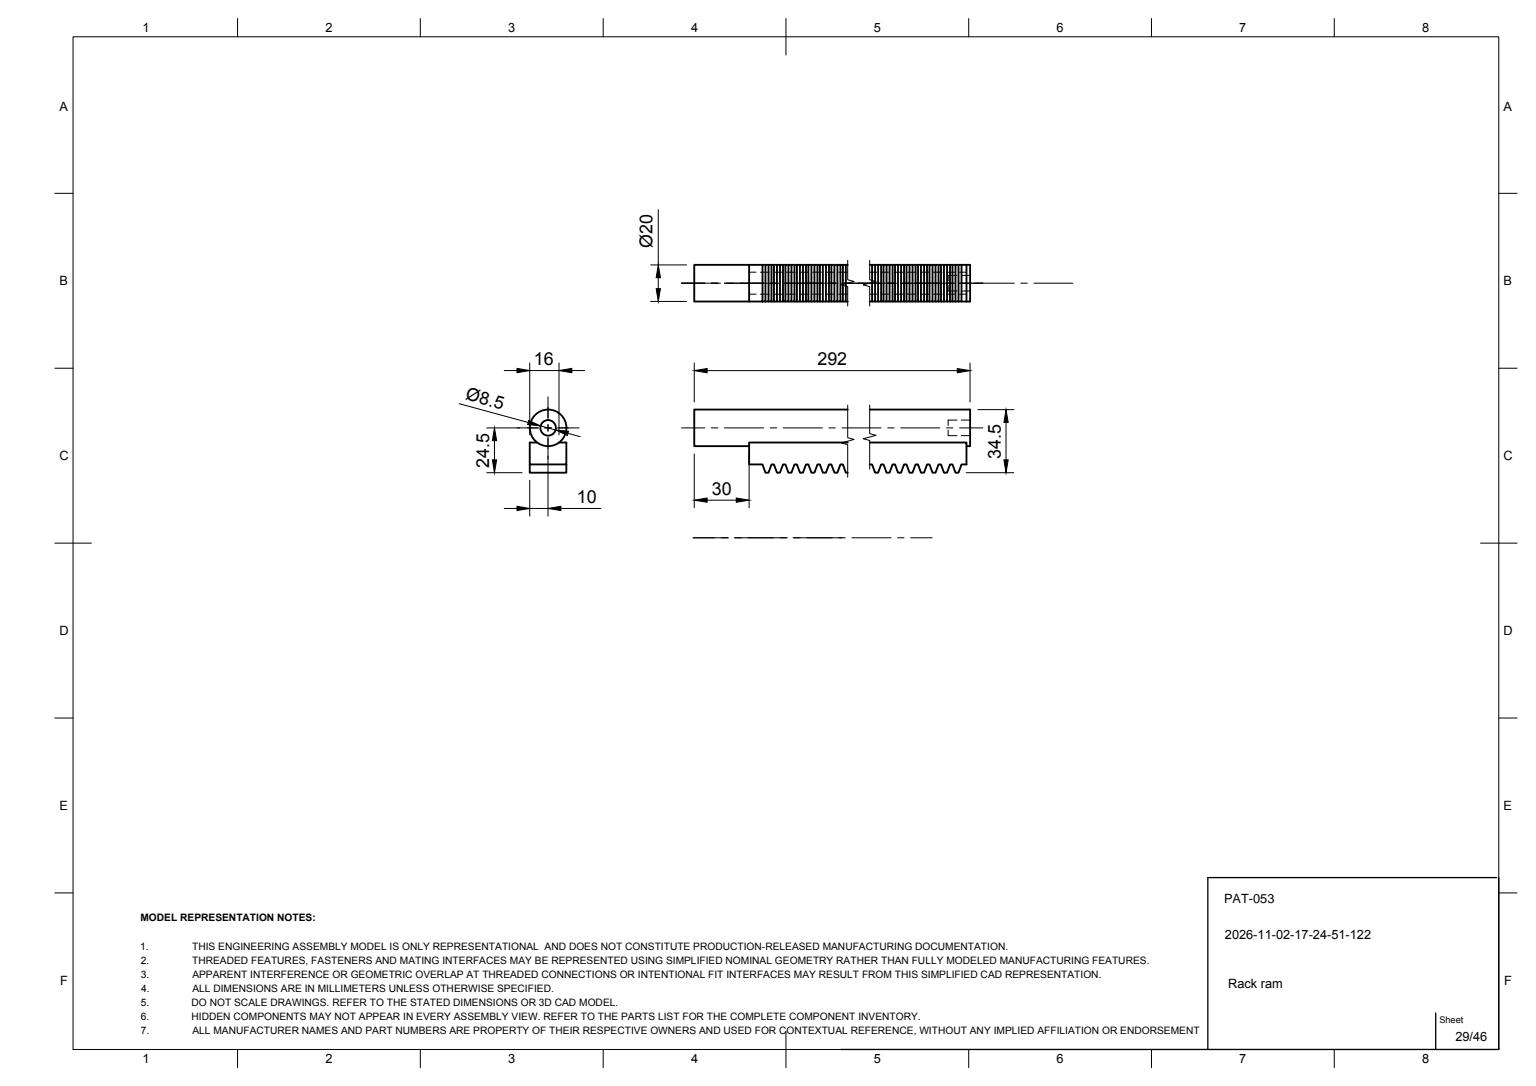
ISO-10303-21;
HEADER;
/* Generated by software containing ST-Developer
 * from STEP Tools, Inc. (www.steptools.com) 
 */

FILE_DESCRIPTION(
/* description */ ('Hand-operated arbor press'),
/* implementation_level */ '2;1');

FILE_NAME(
/* name */ 'Rack ram.step',
/* time_stamp */ '2026-10-28T03:25:25-07:00',
/* author */ (''),
/* organization */ (''),
/* preprocessor_version */ 'ST-DEVELOPER v20.2',
/* originating_system */ 'Autodesk Translation Framework v15.17.0.0',
/* authorisation */ '');

FILE_SCHEMA (('AUTOMOTIVE_DESIGN { 1 0 10303 214 3 1 1 }'));
ENDSEC;

DATA;
#10=MECHANICAL_DESIGN_GEOMETRIC_PRESENTATION_REPRESENTATION('',(#615),#32751);
#524=SHAPE_REPRESENTATION_RELATIONSHIP('SRR','None',#32955,#566);
#566=ADVANCED_BREP_SHAPE_REPRESENTATION('',(#662),#32729);
#615=STYLED_ITEM('',(#33228),#662);
#662=MANIFOLD_SOLID_BREP('Body1',#12514);
#812=FACE_BOUND('',#2561,.T.);
#1004=PLANE('',#13571);
#1005=PLANE('',#13572);
#1006=PLANE('',#13573);
#1007=PLANE('',#13574);
#1008=PLANE('',#13577);
#1009=PLANE('',#13580);
#1010=PLANE('',#13581);
#1011=PLANE('',#13582);
#1012=PLANE('',#13583);
#1013=PLANE('',#13584);
#1014=PLANE('',#13585);
#1015=PLANE('',#13586);
#1016=PLANE('',#13587);
#1017=PLANE('',#13588);
#1018=PLANE('',#13589);
#1019=PLANE('',#13590);
#1020=PLANE('',#13591);
#1021=PLANE('',#13592);
#1022=PLANE('',#13593);
#1023=PLANE('',#13594);
#1024=PLANE('',#13595);
#1025=PLANE('',#13596);
#1026=PLANE('',#13597);
#1027=PLANE('',#13598);
#1028=PLANE('',#13599);
#1029=PLANE('',#13600);
#1030=PLANE('',#13601);
#1031=PLANE('',#13602);
#1032=PLANE('',#13603);
#1033=PLANE('',#13604);
#1034=PLANE('',#13605);
#1035=PLANE('',#13606);
#1036=PLANE('',#13607);
#1037=PLANE('',#13608);
#1038=PLANE('',#13609);
#1039=PLANE('',#13610);
#1040=PLANE('',#13611);
#1041=PLANE('',#13612);
#1042=PLANE('',#13613);
#1043=PLANE('',#13614);
#1044=PLANE('',#13615);
#1045=PLANE('',#13616);
#1046=PLANE('',#13617);
#1047=PLANE('',#13618);
#1048=PLANE('',#13619);
#1049=PLANE('',#13620);
#1050=PLANE('',#13621);
#1051=PLANE('',#13622);
#1052=PLANE('',#13623);
#1053=PLANE('',#13624);
#1054=PLANE('',#13625);
#1055=PLANE('',#13626);
#1056=PLANE('',#13627);
#1057=PLANE('',#13628);
#1058=PLANE('',#13629);
#1059=PLANE('',#13630);
#1060=PLANE('',#13631);
#1061=PLANE('',#13632);
#1062=PLANE('',#13633);
#1063=PLANE('',#13634);
#1064=PLANE('',#13635);
#1065=PLANE('',#13636);
#1066=PLANE('',#13637);
#1067=PLANE('',#13638);
#1068=PLANE('',#13639);
#1069=PLANE('',#13640);
#1070=PLANE('',#13641);
#1071=PLANE('',#13642);
#1072=PLANE('',#13643);
#1073=PLANE('',#13644);
#1074=PLANE('',#13645);
#1075=PLANE('',#13646);
#1076=PLANE('',#13647);
#1077=PLANE('',#13648);
#1078=PLANE('',#13649);
#1079=PLANE('',#13650);
#1080=PLANE('',#13651);
#1081=PLANE('',#13652);
#1082=PLANE('',#13653);
#1083=PLANE('',#13654);
#1084=PLANE('',#13655);
#1085=PLANE('',#13656);
#1086=PLANE('',#13657);
#1087=PLANE('',#13658);
#1088=PLANE('',#13659);
#1089=PLANE('',#13660);
#1090=PLANE('',#13661);
#1091=PLANE('',#13662);
#1092=PLANE('',#13663);
#1093=PLANE('',#13664);
#1094=PLANE('',#13665);
#1095=PLANE('',#13666);
#1096=PLANE('',#13667);
#1097=PLANE('',#13668);
#1098=PLANE('',#13669);
#1099=PLANE('',#13670);
#1100=PLANE('',#13671);
#1101=PLANE('',#13672);
#1102=PLANE('',#13673);
#1103=PLANE('',#13674);
#1104=PLANE('',#13675);
#1105=PLANE('',#13676);
#1106=PLANE('',#13677);
#1107=PLANE('',#13678);
#1108=PLANE('',#13679);
#1109=PLANE('',#13680);
#1110=PLANE('',#13681);
#1111=PLANE('',#13682);
#1112=PLANE('',#13683);
#1113=PLANE('',#13684);
#1114=PLANE('',#13685);
#1115=PLANE('',#13686);
#1116=PLANE('',#13687);
#1117=PLANE('',#13688);
#1118=PLANE('',#13689);
#1119=PLANE('',#13690);
#1120=PLANE('',#13691);
#1121=PLANE('',#13692);
#1122=PLANE('',#13693);
#1123=PLANE('',#13694);
#1124=PLANE('',#13695);
#1125=PLANE('',#13696);
#1126=PLANE('',#13697);
#1127=PLANE('',#13698);
#1128=PLANE('',#13699);
#1129=PLANE('',#13700);
#1130=PLANE('',#13701);
#1131=PLANE('',#13702);
#1132=PLANE('',#13703);
#1133=PLANE('',#13704);
#1134=PLANE('',#13705);
#1135=PLANE('',#13706);
#1136=PLANE('',#13707);
#1137=PLANE('',#13708);
#1138=PLANE('',#13709);
#1139=PLANE('',#13710);
#1140=PLANE('',#13711);
#1141=PLANE('',#13712);
#1142=PLANE('',#13713);
#1143=PLANE('',#13714);
#1144=PLANE('',#13715);
#1145=PLANE('',#13716);
#1146=PLANE('',#13717);
#1147=PLANE('',#13718);
#1148=PLANE('',#13719);
#1149=PLANE('',#13720);
#1150=PLANE('',#13721);
#1151=PLANE('',#13722);
#1152=PLANE('',#13723);
#1153=PLANE('',#13724);
#1154=PLANE('',#13725);
#1155=PLANE('',#13726);
#1156=PLANE('',#13727);
#1157=PLANE('',#13728);
#1158=PLANE('',#13729);
#1159=PLANE('',#13730);
#1160=PLANE('',#13731);
#1161=PLANE('',#13732);
#1162=PLANE('',#13733);
#1163=PLANE('',#13734);
#1164=PLANE('',#13735);
#1165=PLANE('',#13736);
#1166=PLANE('',#13737);
#1167=PLANE('',#13738);
#1168=PLANE('',#13739);
#1169=PLANE('',#13740);
#1170=PLANE('',#13741);
#1171=PLANE('',#13742);
#1172=PLANE('',#13746);
#1173=PLANE('',#13747);
#1576=FACE_OUTER_BOUND('',#2389,.T.);
#1577=FACE_OUTER_BOUND('',#2390,.T.);
#1578=FACE_OUTER_BOUND('',#2391,.T.);
#1579=FACE_OUTER_BOUND('',#2392,.T.);
#1580=FACE_OUTER_BOUND('',#2393,.T.);
#1581=FACE_OUTER_BOUND('',#2394,.T.);
#1582=FACE_OUTER_BOUND('',#2395,.T.);
#1583=FACE_OUTER_BOUND('',#2396,.T.);
#1584=FACE_OUTER_BOUND('',#2397,.T.);
#1585=FACE_OUTER_BOUND('',#2398,.T.);
#1586=FACE_OUTER_BOUND('',#2399,.T.);
#1587=FACE_OUTER_BOUND('',#2400,.T.);
#1588=FACE_OUTER_BOUND('',#2401,.T.);
#1589=FACE_OUTER_BOUND('',#2402,.T.);
#1590=FACE_OUTER_BOUND('',#2403,.T.);
#1591=FACE_OUTER_BOUND('',#2404,.T.);
#1592=FACE_OUTER_BOUND('',#2405,.T.);
#1593=FACE_OUTER_BOUND('',#2406,.T.);
#1594=FACE_OUTER_BOUND('',#2407,.T.);
#1595=FACE_OUTER_BOUND('',#2408,.T.);
#1596=FACE_OUTER_BOUND('',#2409,.T.);
#1597=FACE_OUTER_BOUND('',#2410,.T.);
#1598=FACE_OUTER_BOUND('',#2411,.T.);
#1599=FACE_OUTER_BOUND('',#2412,.T.);
#1600=FACE_OUTER_BOUND('',#2413,.T.);
#1601=FACE_OUTER_BOUND('',#2414,.T.);
#1602=FACE_OUTER_BOUND('',#2415,.T.);
#1603=FACE_OUTER_BOUND('',#2416,.T.);
#1604=FACE_OUTER_BOUND('',#2417,.T.);
#1605=FACE_OUTER_BOUND('',#2418,.T.);
#1606=FACE_OUTER_BOUND('',#2419,.T.);
#1607=FACE_OUTER_BOUND('',#2420,.T.);
#1608=FACE_OUTER_BOUND('',#2421,.T.);
#1609=FACE_OUTER_BOUND('',#2422,.T.);
#1610=FACE_OUTER_BOUND('',#2423,.T.);
#1611=FACE_OUTER_BOUND('',#2424,.T.);
#1612=FACE_OUTER_BOUND('',#2425,.T.);
#1613=FACE_OUTER_BOUND('',#2426,.T.);
#1614=FACE_OUTER_BOUND('',#2427,.T.);
#1615=FACE_OUTER_BOUND('',#2428,.T.);
#1616=FACE_OUTER_BOUND('',#2429,.T.);
#1617=FACE_OUTER_BOUND('',#2430,.T.);
#1618=FACE_OUTER_BOUND('',#2431,.T.);
#1619=FACE_OUTER_BOUND('',#2432,.T.);
#1620=FACE_OUTER_BOUND('',#2433,.T.);
#1621=FACE_OUTER_BOUND('',#2434,.T.);
#1622=FACE_OUTER_BOUND('',#2435,.T.);
#1623=FACE_OUTER_BOUND('',#2436,.T.);
#1624=FACE_OUTER_BOUND('',#2437,.T.);
#1625=FACE_OUTER_BOUND('',#2438,.T.);
#1626=FACE_OUTER_BOUND('',#2439,.T.);
#1627=FACE_OUTER_BOUND('',#2440,.T.);
#1628=FACE_OUTER_BOUND('',#2441,.T.);
#1629=FACE_OUTER_BOUND('',#2442,.T.);
#1630=FACE_OUTER_BOUND('',#2443,.T.);
#1631=FACE_OUTER_BOUND('',#2444,.T.);
#1632=FACE_OUTER_BOUND('',#2445,.T.);
#1633=FACE_OUTER_BOUND('',#2446,.T.);
#1634=FACE_OUTER_BOUND('',#2447,.T.);
#1635=FACE_OUTER_BOUND('',#2448,.T.);
#1636=FACE_OUTER_BOUND('',#2449,.T.);
#1637=FACE_OUTER_BOUND('',#2450,.T.);
#1638=FACE_OUTER_BOUND('',#2451,.T.);
#1639=FACE_OUTER_BOUND('',#2452,.T.);
#1640=FACE_OUTER_BOUND('',#2453,.T.);
#1641=FACE_OUTER_BOUND('',#2454,.T.);
#1642=FACE_OUTER_BOUND('',#2455,.T.);
#1643=FACE_OUTER_BOUND('',#2456,.T.);
#1644=FACE_OUTER_BOUND('',#2457,.T.);
#1645=FACE_OUTER_BOUND('',#2458,.T.);
#1646=FACE_OUTER_BOUND('',#2459,.T.);
#1647=FACE_OUTER_BOUND('',#2460,.T.);
#1648=FACE_OUTER_BOUND('',#2461,.T.);
#1649=FACE_OUTER_BOUND('',#2462,.T.);
#1650=FACE_OUTER_BOUND('',#2463,.T.);
#1651=FACE_OUTER_BOUND('',#2464,.T.);
#1652=FACE_OUTER_BOUND('',#2465,.T.);
#1653=FACE_OUTER_BOUND('',#2466,.T.);
#1654=FACE_OUTER_BOUND('',#2467,.T.);
#1655=FACE_OUTER_BOUND('',#2468,.T.);
#1656=FACE_OUTER_BOUND('',#2469,.T.);
#1657=FACE_OUTER_BOUND('',#2470,.T.);
#1658=FACE_OUTER_BOUND('',#2471,.T.);
#1659=FACE_OUTER_BOUND('',#2472,.T.);
#1660=FACE_OUTER_BOUND('',#2473,.T.);
#1661=FACE_OUTER_BOUND('',#2474,.T.);
#1662=FACE_OUTER_BOUND('',#2475,.T.);
#1663=FACE_OUTER_BOUND('',#2476,.T.);
#1664=FACE_OUTER_BOUND('',#2477,.T.);
#1665=FACE_OUTER_BOUND('',#2478,.T.);
#1666=FACE_OUTER_BOUND('',#2479,.T.);
#1667=FACE_OUTER_BOUND('',#2480,.T.);
#1668=FACE_OUTER_BOUND('',#2481,.T.);
#1669=FACE_OUTER_BOUND('',#2482,.T.);
#1670=FACE_OUTER_BOUND('',#2483,.T.);
#1671=FACE_OUTER_BOUND('',#2484,.T.);
#1672=FACE_OUTER_BOUND('',#2485,.T.);
#1673=FACE_OUTER_BOUND('',#2486,.T.);
#1674=FACE_OUTER_BOUND('',#2487,.T.);
#1675=FACE_OUTER_BOUND('',#2488,.T.);
#1676=FACE_OUTER_BOUND('',#2489,.T.);
#1677=FACE_OUTER_BOUND('',#2490,.T.);
#1678=FACE_OUTER_BOUND('',#2491,.T.);
#1679=FACE_OUTER_BOUND('',#2492,.T.);
#1680=FACE_OUTER_BOUND('',#2493,.T.);
#1681=FACE_OUTER_BOUND('',#2494,.T.);
#1682=FACE_OUTER_BOUND('',#2495,.T.);
#1683=FACE_OUTER_BOUND('',#2496,.T.);
#1684=FACE_OUTER_BOUND('',#2497,.T.);
#1685=FACE_OUTER_BOUND('',#2498,.T.);
#1686=FACE_OUTER_BOUND('',#2499,.T.);
#1687=FACE_OUTER_BOUND('',#2500,.T.);
#1688=FACE_OUTER_BOUND('',#2501,.T.);
#1689=FACE_OUTER_BOUND('',#2502,.T.);
#1690=FACE_OUTER_BOUND('',#2503,.T.);
#1691=FACE_OUTER_BOUND('',#2504,.T.);
#1692=FACE_OUTER_BOUND('',#2505,.T.);
#1693=FACE_OUTER_BOUND('',#2506,.T.);
#1694=FACE_OUTER_BOUND('',#2507,.T.);
#1695=FACE_OUTER_BOUND('',#2508,.T.);
#1696=FACE_OUTER_BOUND('',#2509,.T.);
#1697=FACE_OUTER_BOUND('',#2510,.T.);
#1698=FACE_OUTER_BOUND('',#2511,.T.);
#1699=FACE_OUTER_BOUND('',#2512,.T.);
#1700=FACE_OUTER_BOUND('',#2513,.T.);
#1701=FACE_OUTER_BOUND('',#2514,.T.);
#1702=FACE_OUTER_BOUND('',#2515,.T.);
#1703=FACE_OUTER_BOUND('',#2516,.T.);
#1704=FACE_OUTER_BOUND('',#2517,.T.);
#1705=FACE_OUTER_BOUND('',#2518,.T.);
#1706=FACE_OUTER_BOUND('',#2519,.T.);
#1707=FACE_OUTER_BOUND('',#2520,.T.);
#1708=FACE_OUTER_BOUND('',#2521,.T.);
#1709=FACE_OUTER_BOUND('',#2522,.T.);
#1710=FACE_OUTER_BOUND('',#2523,.T.);
#1711=FACE_OUTER_BOUND('',#2524,.T.);
#1712=FACE_OUTER_BOUND('',#2525,.T.);
#1713=FACE_OUTER_BOUND('',#2526,.T.);
#1714=FACE_OUTER_BOUND('',#2527,.T.);
#1715=FACE_OUTER_BOUND('',#2528,.T.);
#1716=FACE_OUTER_BOUND('',#2529,.T.);
#1717=FACE_OUTER_BOUND('',#2530,.T.);
#1718=FACE_OUTER_BOUND('',#2531,.T.);
#1719=FACE_OUTER_BOUND('',#2532,.T.);
#1720=FACE_OUTER_BOUND('',#2533,.T.);
#1721=FACE_OUTER_BOUND('',#2534,.T.);
#1722=FACE_OUTER_BOUND('',#2535,.T.);
#1723=FACE_OUTER_BOUND('',#2536,.T.);
#1724=FACE_OUTER_BOUND('',#2537,.T.);
#1725=FACE_OUTER_BOUND('',#2538,.T.);
#1726=FACE_OUTER_BOUND('',#2539,.T.);
#1727=FACE_OUTER_BOUND('',#2540,.T.);
#1728=FACE_OUTER_BOUND('',#2541,.T.);
#1729=FACE_OUTER_BOUND('',#2542,.T.);
#1730=FACE_OUTER_BOUND('',#2543,.T.);
#1731=FACE_OUTER_BOUND('',#2544,.T.);
#1732=FACE_OUTER_BOUND('',#2545,.T.);
#1733=FACE_OUTER_BOUND('',#2546,.T.);
#1734=FACE_OUTER_BOUND('',#2547,.T.);
#1735=FACE_OUTER_BOUND('',#2548,.T.);
#1736=FACE_OUTER_BOUND('',#2549,.T.);
#1737=FACE_OUTER_BOUND('',#2550,.T.);
#1738=FACE_OUTER_BOUND('',#2551,.T.);
#1739=FACE_OUTER_BOUND('',#2552,.T.);
#1740=FACE_OUTER_BOUND('',#2553,.T.);
#1741=FACE_OUTER_BOUND('',#2554,.T.);
#1742=FACE_OUTER_BOUND('',#2555,.T.);
#1743=FACE_OUTER_BOUND('',#2556,.T.);
#1744=FACE_OUTER_BOUND('',#2557,.T.);
#1745=FACE_OUTER_BOUND('',#2558,.T.);
#1746=FACE_OUTER_BOUND('',#2559,.T.);
#1747=FACE_OUTER_BOUND('',#2560,.T.);
#2389=EDGE_LOOP('',(#9600,#9601,#9602,#9603));
#2390=EDGE_LOOP('',(#9604));
#2391=EDGE_LOOP('',(#9605,#9606,#9607,#9608));
#2392=EDGE_LOOP('',(#9609,#9610,#9611,#9612));
#2393=EDGE_LOOP('',(#9613,#9614,#9615,#9616,#9617,#9618,#9619));
#2394=EDGE_LOOP('',(#9620,#9621,#9622,#9623,#9624,#9625,#9626));
#2395=EDGE_LOOP('',(#9627,#9628,#9629,#9630));
#2396=EDGE_LOOP('',(#9631,#9632,#9633,#9634));
#2397=EDGE_LOOP('',(#9635,#9636,#9637,#9638));
#2398=EDGE_LOOP('',(#9639,#9640,#9641,#9642));
#2399=EDGE_LOOP('',(#9643,#9644,#9645,#9646));
#2400=EDGE_LOOP('',(#9647,#9648,#9649,#9650));
#2401=EDGE_LOOP('',(#9651,#9652,#9653,#9654));
#2402=EDGE_LOOP('',(#9655,#9656,#9657,#9658));
#2403=EDGE_LOOP('',(#9659,#9660,#9661,#9662));
#2404=EDGE_LOOP('',(#9663,#9664,#9665,#9666));
#2405=EDGE_LOOP('',(#9667,#9668,#9669,#9670));
#2406=EDGE_LOOP('',(#9671,#9672,#9673,#9674));
#2407=EDGE_LOOP('',(#9675,#9676,#9677,#9678));
#2408=EDGE_LOOP('',(#9679,#9680,#9681,#9682));
#2409=EDGE_LOOP('',(#9683,#9684,#9685,#9686));
#2410=EDGE_LOOP('',(#9687,#9688,#9689,#9690));
#2411=EDGE_LOOP('',(#9691,#9692,#9693,#9694));
#2412=EDGE_LOOP('',(#9695,#9696,#9697,#9698));
#2413=EDGE_LOOP('',(#9699,#9700,#9701,#9702));
#2414=EDGE_LOOP('',(#9703,#9704,#9705,#9706));
#2415=EDGE_LOOP('',(#9707,#9708,#9709,#9710));
#2416=EDGE_LOOP('',(#9711,#9712,#9713,#9714));
#2417=EDGE_LOOP('',(#9715,#9716,#9717,#9718));
#2418=EDGE_LOOP('',(#9719,#9720,#9721,#9722));
#2419=EDGE_LOOP('',(#9723,#9724,#9725,#9726));
#2420=EDGE_LOOP('',(#9727,#9728,#9729,#9730));
#2421=EDGE_LOOP('',(#9731,#9732,#9733,#9734));
#2422=EDGE_LOOP('',(#9735,#9736,#9737,#9738));
#2423=EDGE_LOOP('',(#9739,#9740,#9741,#9742));
#2424=EDGE_LOOP('',(#9743,#9744,#9745,#9746));
#2425=EDGE_LOOP('',(#9747,#9748,#9749,#9750));
#2426=EDGE_LOOP('',(#9751,#9752,#9753,#9754));
#2427=EDGE_LOOP('',(#9755,#9756,#9757,#9758));
#2428=EDGE_LOOP('',(#9759,#9760,#9761,#9762));
#2429=EDGE_LOOP('',(#9763,#9764,#9765,#9766));
#2430=EDGE_LOOP('',(#9767,#9768,#9769,#9770));
#2431=EDGE_LOOP('',(#9771,#9772,#9773,#9774));
#2432=EDGE_LOOP('',(#9775,#9776,#9777,#9778));
#2433=EDGE_LOOP('',(#9779,#9780,#9781,#9782));
#2434=EDGE_LOOP('',(#9783,#9784,#9785,#9786));
#2435=EDGE_LOOP('',(#9787,#9788,#9789,#9790));
#2436=EDGE_LOOP('',(#9791,#9792,#9793,#9794));
#2437=EDGE_LOOP('',(#9795,#9796,#9797,#9798));
#2438=EDGE_LOOP('',(#9799,#9800,#9801,#9802));
#2439=EDGE_LOOP('',(#9803,#9804,#9805,#9806));
#2440=EDGE_LOOP('',(#9807,#9808,#9809,#9810));
#2441=EDGE_LOOP('',(#9811,#9812,#9813,#9814));
#2442=EDGE_LOOP('',(#9815,#9816,#9817,#9818));
#2443=EDGE_LOOP('',(#9819,#9820,#9821,#9822));
#2444=EDGE_LOOP('',(#9823,#9824,#9825,#9826));
#2445=EDGE_LOOP('',(#9827,#9828,#9829,#9830));
#2446=EDGE_LOOP('',(#9831,#9832,#9833,#9834));
#2447=EDGE_LOOP('',(#9835,#9836,#9837,#9838));
#2448=EDGE_LOOP('',(#9839,#9840,#9841,#9842));
#2449=EDGE_LOOP('',(#9843,#9844,#9845,#9846));
#2450=EDGE_LOOP('',(#9847,#9848,#9849,#9850));
#2451=EDGE_LOOP('',(#9851,#9852,#9853,#9854));
#2452=EDGE_LOOP('',(#9855,#9856,#9857,#9858));
#2453=EDGE_LOOP('',(#9859,#9860,#9861,#9862));
#2454=EDGE_LOOP('',(#9863,#9864,#9865,#9866));
#2455=EDGE_LOOP('',(#9867,#9868,#9869,#9870));
#2456=EDGE_LOOP('',(#9871,#9872,#9873,#9874));
#2457=EDGE_LOOP('',(#9875,#9876,#9877,#9878));
#2458=EDGE_LOOP('',(#9879,#9880,#9881,#9882));
#2459=EDGE_LOOP('',(#9883,#9884,#9885,#9886));
#2460=EDGE_LOOP('',(#9887,#9888,#9889,#9890));
#2461=EDGE_LOOP('',(#9891,#9892,#9893,#9894));
#2462=EDGE_LOOP('',(#9895,#9896,#9897,#9898));
#2463=EDGE_LOOP('',(#9899,#9900,#9901,#9902));
#2464=EDGE_LOOP('',(#9903,#9904,#9905,#9906));
#2465=EDGE_LOOP('',(#9907,#9908,#9909,#9910));
#2466=EDGE_LOOP('',(#9911,#9912,#9913,#9914));
#2467=EDGE_LOOP('',(#9915,#9916,#9917,#9918));
#2468=EDGE_LOOP('',(#9919,#9920,#9921,#9922));
#2469=EDGE_LOOP('',(#9923,#9924,#9925,#9926));
#2470=EDGE_LOOP('',(#9927,#9928,#9929,#9930));
#2471=EDGE_LOOP('',(#9931,#9932,#9933,#9934));
#2472=EDGE_LOOP('',(#9935,#9936,#9937,#9938));
#2473=EDGE_LOOP('',(#9939,#9940,#9941,#9942));
#2474=EDGE_LOOP('',(#9943,#9944,#9945,#9946));
#2475=EDGE_LOOP('',(#9947,#9948,#9949,#9950));
#2476=EDGE_LOOP('',(#9951,#9952,#9953,#9954));
#2477=EDGE_LOOP('',(#9955,#9956,#9957,#9958));
#2478=EDGE_LOOP('',(#9959,#9960,#9961,#9962));
#2479=EDGE_LOOP('',(#9963,#9964,#9965,#9966));
#2480=EDGE_LOOP('',(#9967,#9968,#9969,#9970));
#2481=EDGE_LOOP('',(#9971,#9972,#9973,#9974));
#2482=EDGE_LOOP('',(#9975,#9976,#9977,#9978));
#2483=EDGE_LOOP('',(#9979,#9980,#9981,#9982));
#2484=EDGE_LOOP('',(#9983,#9984,#9985,#9986));
#2485=EDGE_LOOP('',(#9987,#9988,#9989,#9990));
#2486=EDGE_LOOP('',(#9991,#9992,#9993,#9994));
#2487=EDGE_LOOP('',(#9995,#9996,#9997,#9998));
#2488=EDGE_LOOP('',(#9999,#10000,#10001,#10002));
#2489=EDGE_LOOP('',(#10003,#10004,#10005,#10006));
#2490=EDGE_LOOP('',(#10007,#10008,#10009,#10010));
#2491=EDGE_LOOP('',(#10011,#10012,#10013,#10014));
#2492=EDGE_LOOP('',(#10015,#10016,#10017,#10018));
#2493=EDGE_LOOP('',(#10019,#10020,#10021,#10022));
#2494=EDGE_LOOP('',(#10023,#10024,#10025,#10026));
#2495=EDGE_LOOP('',(#10027,#10028,#10029,#10030));
#2496=EDGE_LOOP('',(#10031,#10032,#10033,#10034));
#2497=EDGE_LOOP('',(#10035,#10036,#10037,#10038));
#2498=EDGE_LOOP('',(#10039,#10040,#10041,#10042));
#2499=EDGE_LOOP('',(#10043,#10044,#10045,#10046));
#2500=EDGE_LOOP('',(#10047,#10048,#10049,#10050));
#2501=EDGE_LOOP('',(#10051,#10052,#10053,#10054));
#2502=EDGE_LOOP('',(#10055,#10056,#10057,#10058));
#2503=EDGE_LOOP('',(#10059,#10060,#10061,#10062));
#2504=EDGE_LOOP('',(#10063,#10064,#10065,#10066));
#2505=EDGE_LOOP('',(#10067,#10068,#10069,#10070));
#2506=EDGE_LOOP('',(#10071,#10072,#10073,#10074));
#2507=EDGE_LOOP('',(#10075,#10076,#10077,#10078));
#2508=EDGE_LOOP('',(#10079,#10080,#10081,#10082));
#2509=EDGE_LOOP('',(#10083,#10084,#10085,#10086));
#2510=EDGE_LOOP('',(#10087,#10088,#10089,#10090));
#2511=EDGE_LOOP('',(#10091,#10092,#10093,#10094));
#2512=EDGE_LOOP('',(#10095,#10096,#10097,#10098));
#2513=EDGE_LOOP('',(#10099,#10100,#10101,#10102));
#2514=EDGE_LOOP('',(#10103,#10104,#10105,#10106));
#2515=EDGE_LOOP('',(#10107,#10108,#10109,#10110));
#2516=EDGE_LOOP('',(#10111,#10112,#10113,#10114));
#2517=EDGE_LOOP('',(#10115,#10116,#10117,#10118));
#2518=EDGE_LOOP('',(#10119,#10120,#10121,#10122));
#2519=EDGE_LOOP('',(#10123,#10124,#10125,#10126));
#2520=EDGE_LOOP('',(#10127,#10128,#10129,#10130));
#2521=EDGE_LOOP('',(#10131,#10132,#10133,#10134));
#2522=EDGE_LOOP('',(#10135,#10136,#10137,#10138));
#2523=EDGE_LOOP('',(#10139,#10140,#10141,#10142));
#2524=EDGE_LOOP('',(#10143,#10144,#10145,#10146));
#2525=EDGE_LOOP('',(#10147,#10148,#10149,#10150));
#2526=EDGE_LOOP('',(#10151,#10152,#10153,#10154));
#2527=EDGE_LOOP('',(#10155,#10156,#10157,#10158));
#2528=EDGE_LOOP('',(#10159,#10160,#10161,#10162));
#2529=EDGE_LOOP('',(#10163,#10164,#10165,#10166));
#2530=EDGE_LOOP('',(#10167,#10168,#10169,#10170));
#2531=EDGE_LOOP('',(#10171,#10172,#10173,#10174));
#2532=EDGE_LOOP('',(#10175,#10176,#10177,#10178));
#2533=EDGE_LOOP('',(#10179,#10180,#10181,#10182));
#2534=EDGE_LOOP('',(#10183,#10184,#10185,#10186));
#2535=EDGE_LOOP('',(#10187,#10188,#10189,#10190));
#2536=EDGE_LOOP('',(#10191,#10192,#10193,#10194));
#2537=EDGE_LOOP('',(#10195,#10196,#10197,#10198));
#2538=EDGE_LOOP('',(#10199,#10200,#10201,#10202));
#2539=EDGE_LOOP('',(#10203,#10204,#10205,#10206));
#2540=EDGE_LOOP('',(#10207,#10208,#10209,#10210));
#2541=EDGE_LOOP('',(#10211,#10212,#10213,#10214));
#2542=EDGE_LOOP('',(#10215,#10216,#10217,#10218));
#2543=EDGE_LOOP('',(#10219,#10220,#10221,#10222));
#2544=EDGE_LOOP('',(#10223,#10224,#10225,#10226));
#2545=EDGE_LOOP('',(#10227,#10228,#10229,#10230));
#2546=EDGE_LOOP('',(#10231,#10232,#10233,#10234));
#2547=EDGE_LOOP('',(#10235,#10236,#10237,#10238));
#2548=EDGE_LOOP('',(#10239,#10240,#10241,#10242));
#2549=EDGE_LOOP('',(#10243,#10244,#10245,#10246));
#2550=EDGE_LOOP('',(#10247,#10248,#10249,#10250));
#2551=EDGE_LOOP('',(#10251,#10252,#10253,#10254));
#2552=EDGE_LOOP('',(#10255,#10256,#10257,#10258));
#2553=EDGE_LOOP('',(#10259,#10260,#10261,#10262));
#2554=EDGE_LOOP('',(#10263,#10264,#10265,#10266));
#2555=EDGE_LOOP('',(#10267,#10268,#10269,#10270));
#2556=EDGE_LOOP('',(#10271,#10272,#10273,#10274,#10275,#10276,#10277,#10278,
#10279,#10280,#10281,#10282,#10283,#10284,#10285,#10286,#10287,#10288,#10289,
#10290,#10291,#10292,#10293,#10294,#10295,#10296,#10297,#10298,#10299,#10300,
#10301,#10302,#10303,#10304,#10305,#10306,#10307,#10308,#10309,#10310,#10311,
#10312,#10313,#10314,#10315,#10316,#10317,#10318,#10319,#10320,#10321,#10322,
#10323,#10324,#10325,#10326,#10327,#10328,#10329,#10330,#10331,#10332,#10333,
#10334,#10335,#10336,#10337,#10338,#10339,#10340,#10341,#10342,#10343,#10344,
#10345,#10346,#10347,#10348,#10349,#10350,#10351,#10352,#10353,#10354,#10355,
#10356,#10357,#10358,#10359,#10360,#10361,#10362,#10363,#10364,#10365,#10366,
#10367,#10368,#10369,#10370,#10371,#10372,#10373,#10374,#10375,#10376,#10377,
#10378,#10379,#10380,#10381,#10382,#10383,#10384,#10385,#10386,#10387,#10388,
#10389,#10390,#10391,#10392,#10393,#10394,#10395,#10396,#10397,#10398,#10399,
#10400,#10401,#10402,#10403,#10404,#10405,#10406,#10407,#10408,#10409,#10410,
#10411,#10412,#10413,#10414,#10415,#10416,#10417,#10418,#10419,#10420,#10421,
#10422,#10423,#10424,#10425,#10426,#10427,#10428,#10429,#10430,#10431,#10432,
#10433,#10434));
#2557=EDGE_LOOP('',(#10435,#10436,#10437,#10438,#10439,#10440,#10441,#10442,
#10443,#10444,#10445,#10446,#10447,#10448,#10449,#10450,#10451,#10452,#10453,
#10454,#10455,#10456,#10457,#10458,#10459,#10460,#10461,#10462,#10463,#10464,
#10465,#10466,#10467,#10468,#10469,#10470,#10471,#10472,#10473,#10474,#10475,
#10476,#10477,#10478,#10479,#10480,#10481,#10482,#10483,#10484,#10485,#10486,
#10487,#10488,#10489,#10490,#10491,#10492,#10493,#10494,#10495,#10496,#10497,
#10498,#10499,#10500,#10501,#10502,#10503,#10504,#10505,#10506,#10507,#10508,
#10509,#10510,#10511,#10512,#10513,#10514,#10515,#10516,#10517,#10518,#10519,
#10520,#10521,#10522,#10523,#10524,#10525,#10526,#10527,#10528,#10529,#10530,
#10531,#10532,#10533,#10534,#10535,#10536,#10537,#10538,#10539,#10540,#10541,
#10542,#10543,#10544,#10545,#10546,#10547,#10548,#10549,#10550,#10551,#10552,
#10553,#10554,#10555,#10556,#10557,#10558,#10559,#10560,#10561,#10562,#10563,
#10564,#10565,#10566,#10567,#10568,#10569,#10570,#10571,#10572,#10573,#10574,
#10575,#10576,#10577,#10578,#10579,#10580,#10581,#10582,#10583,#10584,#10585,
#10586,#10587,#10588,#10589,#10590,#10591,#10592,#10593,#10594,#10595,#10596,
#10597,#10598));
#2558=EDGE_LOOP('',(#10599,#10600,#10601,#10602,#10603,#10604,#10605,#10606,
#10607,#10608,#10609,#10610));
#2559=EDGE_LOOP('',(#10611));
#2560=EDGE_LOOP('',(#10612));
#2561=EDGE_LOOP('',(#10613));
#3194=LINE('',#19320,#4365);
#3195=LINE('',#19326,#4366);
#3196=LINE('',#19328,#4367);
#3197=LINE('',#19330,#4368);
#3198=LINE('',#19331,#4369);
#3199=LINE('',#19335,#4370);
#3200=LINE('',#19337,#4371);
#3201=LINE('',#19339,#4372);
#3202=LINE('',#19340,#4373);
#3203=LINE('',#19345,#4374);
#3204=LINE('',#19347,#4375);
#3205=LINE('',#19348,#4376);
#3206=LINE('',#19354,#4377);
#3207=LINE('',#19356,#4378);
#3208=LINE('',#19357,#4379);
#3209=LINE('',#19361,#4380);
#3210=LINE('',#19363,#4381);
#3211=LINE('',#19364,#4382);
#3212=LINE('',#19367,#4383);
#3213=LINE('',#19369,#4384);
#3214=LINE('',#19370,#4385);
#3215=LINE('',#19373,#4386);
#3216=LINE('',#19375,#4387);
#3217=LINE('',#19376,#4388);
#3218=LINE('',#19379,#4389);
#3219=LINE('',#19381,#4390);
#3220=LINE('',#19382,#4391);
#3221=LINE('',#19385,#4392);
#3222=LINE('',#19387,#4393);
#3223=LINE('',#19388,#4394);
#3224=LINE('',#19391,#4395);
#3225=LINE('',#19393,#4396);
#3226=LINE('',#19394,#4397);
#3227=LINE('',#19397,#4398);
#3228=LINE('',#19399,#4399);
#3229=LINE('',#19400,#4400);
#3230=LINE('',#19403,#4401);
#3231=LINE('',#19405,#4402);
#3232=LINE('',#19406,#4403);
#3233=LINE('',#19409,#4404);
#3234=LINE('',#19411,#4405);
#3235=LINE('',#19412,#4406);
#3236=LINE('',#19415,#4407);
#3237=LINE('',#19417,#4408);
#3238=LINE('',#19418,#4409);
#3239=LINE('',#19421,#4410);
#3240=LINE('',#19423,#4411);
#3241=LINE('',#19424,#4412);
#3242=LINE('',#19427,#4413);
#3243=LINE('',#19429,#4414);
#3244=LINE('',#19430,#4415);
#3245=LINE('',#19433,#4416);
#3246=LINE('',#19435,#4417);
#3247=LINE('',#19436,#4418);
#3248=LINE('',#19439,#4419);
#3249=LINE('',#19441,#4420);
#3250=LINE('',#19442,#4421);
#3251=LINE('',#19445,#4422);
#3252=LINE('',#19447,#4423);
#3253=LINE('',#19448,#4424);
#3254=LINE('',#19451,#4425);
#3255=LINE('',#19453,#4426);
#3256=LINE('',#19454,#4427);
#3257=LINE('',#19457,#4428);
#3258=LINE('',#19459,#4429);
#3259=LINE('',#19460,#4430);
#3260=LINE('',#19463,#4431);
#3261=LINE('',#19465,#4432);
#3262=LINE('',#19466,#4433);
#3263=LINE('',#19469,#4434);
#3264=LINE('',#19471,#4435);
#3265=LINE('',#19472,#4436);
#3266=LINE('',#19475,#4437);
#3267=LINE('',#19477,#4438);
#3268=LINE('',#19478,#4439);
#3269=LINE('',#19481,#4440);
#3270=LINE('',#19483,#4441);
#3271=LINE('',#19484,#4442);
#3272=LINE('',#19487,#4443);
#3273=LINE('',#19489,#4444);
#3274=LINE('',#19490,#4445);
#3275=LINE('',#19493,#4446);
#3276=LINE('',#19495,#4447);
#3277=LINE('',#19496,#4448);
#3278=LINE('',#19499,#4449);
#3279=LINE('',#19501,#4450);
#3280=LINE('',#19502,#4451);
#3281=LINE('',#19505,#4452);
#3282=LINE('',#19507,#4453);
#3283=LINE('',#19508,#4454);
#3284=LINE('',#19511,#4455);
#3285=LINE('',#19513,#4456);
#3286=LINE('',#19514,#4457);
#3287=LINE('',#19517,#4458);
#3288=LINE('',#19519,#4459);
#3289=LINE('',#19520,#4460);
#3290=LINE('',#19523,#4461);
#3291=LINE('',#19525,#4462);
#3292=LINE('',#19526,#4463);
#3293=LINE('',#19529,#4464);
#3294=LINE('',#19531,#4465);
#3295=LINE('',#19532,#4466);
#3296=LINE('',#19535,#4467);
#3297=LINE('',#19537,#4468);
#3298=LINE('',#19538,#4469);
#3299=LINE('',#19541,#4470);
#3300=LINE('',#19543,#4471);
#3301=LINE('',#19544,#4472);
#3302=LINE('',#19547,#4473);
#3303=LINE('',#19549,#4474);
#3304=LINE('',#19550,#4475);
#3305=LINE('',#19553,#4476);
#3306=LINE('',#19555,#4477);
#3307=LINE('',#19556,#4478);
#3308=LINE('',#19559,#4479);
#3309=LINE('',#19561,#4480);
#3310=LINE('',#19562,#4481);
#3311=LINE('',#19565,#4482);
#3312=LINE('',#19567,#4483);
#3313=LINE('',#19568,#4484);
#3314=LINE('',#19571,#4485);
#3315=LINE('',#19573,#4486);
#3316=LINE('',#19574,#4487);
#3317=LINE('',#19577,#4488);
#3318=LINE('',#19579,#4489);
#3319=LINE('',#19580,#4490);
#3320=LINE('',#19583,#4491);
#3321=LINE('',#19585,#4492);
#3322=LINE('',#19586,#4493);
#3323=LINE('',#19589,#4494);
#3324=LINE('',#19591,#4495);
#3325=LINE('',#19592,#4496);
#3326=LINE('',#19595,#4497);
#3327=LINE('',#19597,#4498);
#3328=LINE('',#19598,#4499);
#3329=LINE('',#19601,#4500);
#3330=LINE('',#19603,#4501);
#3331=LINE('',#19604,#4502);
#3332=LINE('',#19607,#4503);
#3333=LINE('',#19609,#4504);
#3334=LINE('',#19610,#4505);
#3335=LINE('',#19613,#4506);
#3336=LINE('',#19615,#4507);
#3337=LINE('',#19616,#4508);
#3338=LINE('',#19619,#4509);
#3339=LINE('',#19621,#4510);
#3340=LINE('',#19622,#4511);
#3341=LINE('',#19625,#4512);
#3342=LINE('',#19627,#4513);
#3343=LINE('',#19628,#4514);
#3344=LINE('',#19631,#4515);
#3345=LINE('',#19633,#4516);
#3346=LINE('',#19634,#4517);
#3347=LINE('',#19637,#4518);
#3348=LINE('',#19639,#4519);
#3349=LINE('',#19640,#4520);
#3350=LINE('',#19643,#4521);
#3351=LINE('',#19645,#4522);
#3352=LINE('',#19646,#4523);
#3353=LINE('',#19649,#4524);
#3354=LINE('',#19651,#4525);
#3355=LINE('',#19652,#4526);
#3356=LINE('',#19655,#4527);
#3357=LINE('',#19657,#4528);
#3358=LINE('',#19658,#4529);
#3359=LINE('',#19661,#4530);
#3360=LINE('',#19663,#4531);
#3361=LINE('',#19664,#4532);
#3362=LINE('',#19667,#4533);
#3363=LINE('',#19669,#4534);
#3364=LINE('',#19670,#4535);
#3365=LINE('',#19673,#4536);
#3366=LINE('',#19675,#4537);
#3367=LINE('',#19676,#4538);
#3368=LINE('',#19679,#4539);
#3369=LINE('',#19681,#4540);
#3370=LINE('',#19682,#4541);
#3371=LINE('',#19685,#4542);
#3372=LINE('',#19687,#4543);
#3373=LINE('',#19688,#4544);
#3374=LINE('',#19691,#4545);
#3375=LINE('',#19693,#4546);
#3376=LINE('',#19694,#4547);
#3377=LINE('',#19697,#4548);
#3378=LINE('',#19699,#4549);
#3379=LINE('',#19700,#4550);
#3380=LINE('',#19703,#4551);
#3381=LINE('',#19705,#4552);
#3382=LINE('',#19706,#4553);
#3383=LINE('',#19709,#4554);
#3384=LINE('',#19711,#4555);
#3385=LINE('',#19712,#4556);
#3386=LINE('',#19715,#4557);
#3387=LINE('',#19717,#4558);
#3388=LINE('',#19718,#4559);
#3389=LINE('',#19721,#4560);
#3390=LINE('',#19723,#4561);
#3391=LINE('',#19724,#4562);
#3392=LINE('',#19727,#4563);
#3393=LINE('',#19729,#4564);
#3394=LINE('',#19730,#4565);
#3395=LINE('',#19733,#4566);
#3396=LINE('',#19735,#4567);
#3397=LINE('',#19736,#4568);
#3398=LINE('',#19739,#4569);
#3399=LINE('',#19741,#4570);
#3400=LINE('',#19742,#4571);
#3401=LINE('',#19745,#4572);
#3402=LINE('',#19747,#4573);
#3403=LINE('',#19748,#4574);
#3404=LINE('',#19751,#4575);
#3405=LINE('',#19753,#4576);
#3406=LINE('',#19754,#4577);
#3407=LINE('',#19757,#4578);
#3408=LINE('',#19759,#4579);
#3409=LINE('',#19760,#4580);
#3410=LINE('',#19763,#4581);
#3411=LINE('',#19765,#4582);
#3412=LINE('',#19766,#4583);
#3413=LINE('',#19769,#4584);
#3414=LINE('',#19771,#4585);
#3415=LINE('',#19772,#4586);
#3416=LINE('',#19775,#4587);
#3417=LINE('',#19777,#4588);
#3418=LINE('',#19778,#4589);
#3419=LINE('',#19781,#4590);
#3420=LINE('',#19783,#4591);
#3421=LINE('',#19784,#4592);
#3422=LINE('',#19787,#4593);
#3423=LINE('',#19789,#4594);
#3424=LINE('',#19790,#4595);
#3425=LINE('',#19793,#4596);
#3426=LINE('',#19795,#4597);
#3427=LINE('',#19796,#4598);
#3428=LINE('',#19799,#4599);
#3429=LINE('',#19801,#4600);
#3430=LINE('',#19802,#4601);
#3431=LINE('',#19805,#4602);
#3432=LINE('',#19807,#4603);
#3433=LINE('',#19808,#4604);
#3434=LINE('',#19811,#4605);
#3435=LINE('',#19813,#4606);
#3436=LINE('',#19814,#4607);
#3437=LINE('',#19817,#4608);
#3438=LINE('',#19819,#4609);
#3439=LINE('',#19820,#4610);
#3440=LINE('',#19823,#4611);
#3441=LINE('',#19825,#4612);
#3442=LINE('',#19826,#4613);
#3443=LINE('',#19829,#4614);
#3444=LINE('',#19831,#4615);
#3445=LINE('',#19832,#4616);
#3446=LINE('',#19835,#4617);
#3447=LINE('',#19837,#4618);
#3448=LINE('',#19838,#4619);
#3449=LINE('',#19841,#4620);
#3450=LINE('',#19843,#4621);
#3451=LINE('',#19844,#4622);
#3452=LINE('',#19847,#4623);
#3453=LINE('',#19849,#4624);
#3454=LINE('',#19850,#4625);
#3455=LINE('',#19853,#4626);
#3456=LINE('',#19855,#4627);
#3457=LINE('',#19856,#4628);
#3458=LINE('',#19859,#4629);
#3459=LINE('',#19861,#4630);
#3460=LINE('',#19862,#4631);
#3461=LINE('',#19865,#4632);
#3462=LINE('',#19867,#4633);
#3463=LINE('',#19868,#4634);
#3464=LINE('',#19871,#4635);
#3465=LINE('',#19873,#4636);
#3466=LINE('',#19874,#4637);
#3467=LINE('',#19877,#4638);
#3468=LINE('',#19879,#4639);
#3469=LINE('',#19880,#4640);
#3470=LINE('',#19883,#4641);
#3471=LINE('',#19885,#4642);
#3472=LINE('',#19886,#4643);
#3473=LINE('',#19889,#4644);
#3474=LINE('',#19891,#4645);
#3475=LINE('',#19892,#4646);
#3476=LINE('',#19895,#4647);
#3477=LINE('',#19897,#4648);
#3478=LINE('',#19898,#4649);
#3479=LINE('',#19901,#4650);
#3480=LINE('',#19903,#4651);
#3481=LINE('',#19904,#4652);
#3482=LINE('',#19907,#4653);
#3483=LINE('',#19909,#4654);
#3484=LINE('',#19910,#4655);
#3485=LINE('',#19913,#4656);
#3486=LINE('',#19915,#4657);
#3487=LINE('',#19916,#4658);
#3488=LINE('',#19919,#4659);
#3489=LINE('',#19921,#4660);
#3490=LINE('',#19922,#4661);
#3491=LINE('',#19925,#4662);
#3492=LINE('',#19927,#4663);
#3493=LINE('',#19928,#4664);
#3494=LINE('',#19931,#4665);
#3495=LINE('',#19933,#4666);
#3496=LINE('',#19934,#4667);
#3497=LINE('',#19937,#4668);
#3498=LINE('',#19939,#4669);
#3499=LINE('',#19940,#4670);
#3500=LINE('',#19943,#4671);
#3501=LINE('',#19945,#4672);
#3502=LINE('',#19946,#4673);
#3503=LINE('',#19949,#4674);
#3504=LINE('',#19951,#4675);
#3505=LINE('',#19952,#4676);
#3506=LINE('',#19955,#4677);
#3507=LINE('',#19957,#4678);
#3508=LINE('',#19958,#4679);
#3509=LINE('',#19961,#4680);
#3510=LINE('',#19963,#4681);
#3511=LINE('',#19964,#4682);
#3512=LINE('',#19967,#4683);
#3513=LINE('',#19969,#4684);
#3514=LINE('',#19970,#4685);
#3515=LINE('',#19973,#4686);
#3516=LINE('',#19975,#4687);
#3517=LINE('',#19976,#4688);
#3518=LINE('',#19979,#4689);
#3519=LINE('',#19981,#4690);
#3520=LINE('',#19982,#4691);
#3521=LINE('',#19985,#4692);
#3522=LINE('',#19987,#4693);
#3523=LINE('',#19988,#4694);
#3524=LINE('',#19991,#4695);
#3525=LINE('',#19993,#4696);
#3526=LINE('',#19994,#4697);
#3527=LINE('',#19997,#4698);
#3528=LINE('',#19999,#4699);
#3529=LINE('',#20000,#4700);
#3530=LINE('',#20003,#4701);
#3531=LINE('',#20005,#4702);
#3532=LINE('',#20006,#4703);
#3533=LINE('',#20009,#4704);
#3534=LINE('',#20011,#4705);
#3535=LINE('',#20012,#4706);
#3536=LINE('',#20015,#4707);
#3537=LINE('',#20017,#4708);
#3538=LINE('',#20018,#4709);
#3539=LINE('',#20021,#4710);
#3540=LINE('',#20023,#4711);
#3541=LINE('',#20024,#4712);
#3542=LINE('',#20027,#4713);
#3543=LINE('',#20029,#4714);
#3544=LINE('',#20030,#4715);
#3545=LINE('',#20033,#4716);
#3546=LINE('',#20035,#4717);
#3547=LINE('',#20036,#4718);
#3548=LINE('',#20039,#4719);
#3549=LINE('',#20041,#4720);
#3550=LINE('',#20042,#4721);
#3551=LINE('',#20045,#4722);
#3552=LINE('',#20047,#4723);
#3553=LINE('',#20048,#4724);
#3554=LINE('',#20051,#4725);
#3555=LINE('',#20053,#4726);
#3556=LINE('',#20054,#4727);
#3557=LINE('',#20057,#4728);
#3558=LINE('',#20059,#4729);
#3559=LINE('',#20060,#4730);
#3560=LINE('',#20063,#4731);
#3561=LINE('',#20065,#4732);
#3562=LINE('',#20066,#4733);
#3563=LINE('',#20069,#4734);
#3564=LINE('',#20071,#4735);
#3565=LINE('',#20072,#4736);
#3566=LINE('',#20075,#4737);
#3567=LINE('',#20077,#4738);
#3568=LINE('',#20078,#4739);
#3569=LINE('',#20081,#4740);
#3570=LINE('',#20083,#4741);
#3571=LINE('',#20084,#4742);
#3572=LINE('',#20087,#4743);
#3573=LINE('',#20089,#4744);
#3574=LINE('',#20090,#4745);
#3575=LINE('',#20093,#4746);
#3576=LINE('',#20095,#4747);
#3577=LINE('',#20096,#4748);
#3578=LINE('',#20099,#4749);
#3579=LINE('',#20101,#4750);
#3580=LINE('',#20102,#4751);
#3581=LINE('',#20105,#4752);
#3582=LINE('',#20107,#4753);
#3583=LINE('',#20108,#4754);
#3584=LINE('',#20111,#4755);
#3585=LINE('',#20113,#4756);
#3586=LINE('',#20114,#4757);
#3587=LINE('',#20117,#4758);
#3588=LINE('',#20119,#4759);
#3589=LINE('',#20120,#4760);
#3590=LINE('',#20123,#4761);
#3591=LINE('',#20125,#4762);
#3592=LINE('',#20126,#4763);
#3593=LINE('',#20129,#4764);
#3594=LINE('',#20131,#4765);
#3595=LINE('',#20132,#4766);
#3596=LINE('',#20135,#4767);
#3597=LINE('',#20137,#4768);
#3598=LINE('',#20138,#4769);
#3599=LINE('',#20141,#4770);
#3600=LINE('',#20143,#4771);
#3601=LINE('',#20144,#4772);
#3602=LINE('',#20147,#4773);
#3603=LINE('',#20149,#4774);
#3604=LINE('',#20150,#4775);
#3605=LINE('',#20153,#4776);
#3606=LINE('',#20155,#4777);
#3607=LINE('',#20156,#4778);
#3608=LINE('',#20159,#4779);
#3609=LINE('',#20161,#4780);
#3610=LINE('',#20162,#4781);
#3611=LINE('',#20165,#4782);
#3612=LINE('',#20167,#4783);
#3613=LINE('',#20168,#4784);
#3614=LINE('',#20171,#4785);
#3615=LINE('',#20173,#4786);
#3616=LINE('',#20174,#4787);
#3617=LINE('',#20177,#4788);
#3618=LINE('',#20179,#4789);
#3619=LINE('',#20180,#4790);
#3620=LINE('',#20183,#4791);
#3621=LINE('',#20185,#4792);
#3622=LINE('',#20186,#4793);
#3623=LINE('',#20189,#4794);
#3624=LINE('',#20191,#4795);
#3625=LINE('',#20192,#4796);
#3626=LINE('',#20195,#4797);
#3627=LINE('',#20197,#4798);
#3628=LINE('',#20198,#4799);
#3629=LINE('',#20201,#4800);
#3630=LINE('',#20203,#4801);
#3631=LINE('',#20204,#4802);
#3632=LINE('',#20207,#4803);
#3633=LINE('',#20209,#4804);
#3634=LINE('',#20210,#4805);
#3635=LINE('',#20213,#4806);
#3636=LINE('',#20215,#4807);
#3637=LINE('',#20216,#4808);
#3638=LINE('',#20219,#4809);
#3639=LINE('',#20221,#4810);
#3640=LINE('',#20222,#4811);
#3641=LINE('',#20225,#4812);
#3642=LINE('',#20227,#4813);
#3643=LINE('',#20228,#4814);
#3644=LINE('',#20231,#4815);
#3645=LINE('',#20233,#4816);
#3646=LINE('',#20234,#4817);
#3647=LINE('',#20237,#4818);
#3648=LINE('',#20239,#4819);
#3649=LINE('',#20240,#4820);
#3650=LINE('',#20243,#4821);
#3651=LINE('',#20245,#4822);
#3652=LINE('',#20246,#4823);
#3653=LINE('',#20249,#4824);
#3654=LINE('',#20251,#4825);
#3655=LINE('',#20252,#4826);
#3656=LINE('',#20255,#4827);
#3657=LINE('',#20257,#4828);
#3658=LINE('',#20258,#4829);
#3659=LINE('',#20261,#4830);
#3660=LINE('',#20263,#4831);
#3661=LINE('',#20264,#4832);
#3662=LINE('',#20267,#4833);
#3663=LINE('',#20269,#4834);
#3664=LINE('',#20270,#4835);
#3665=LINE('',#20273,#4836);
#3666=LINE('',#20275,#4837);
#3667=LINE('',#20276,#4838);
#3668=LINE('',#20279,#4839);
#3669=LINE('',#20281,#4840);
#3670=LINE('',#20282,#4841);
#3671=LINE('',#20285,#4842);
#3672=LINE('',#20287,#4843);
#3673=LINE('',#20288,#4844);
#3674=LINE('',#20291,#4845);
#3675=LINE('',#20293,#4846);
#3676=LINE('',#20294,#4847);
#3677=LINE('',#20297,#4848);
#3678=LINE('',#20299,#4849);
#3679=LINE('',#20300,#4850);
#3680=LINE('',#20303,#4851);
#3681=LINE('',#20305,#4852);
#3682=LINE('',#20306,#4853);
#3683=LINE('',#20309,#4854);
#3684=LINE('',#20311,#4855);
#3685=LINE('',#20312,#4856);
#3686=LINE('',#20315,#4857);
#3687=LINE('',#20317,#4858);
#3688=LINE('',#20318,#4859);
#3689=LINE('',#20320,#4860);
#3690=LINE('',#20321,#4861);
#3691=LINE('',#20327,#4862);
#3692=LINE('',#20329,#4863);
#4365=VECTOR('',#15667,0.425);
#4366=VECTOR('',#15674,1.);
#4367=VECTOR('',#15675,1.);
#4368=VECTOR('',#15676,1.);
#4369=VECTOR('',#15677,1.);
#4370=VECTOR('',#15680,1.);
#4371=VECTOR('',#15681,1.);
#4372=VECTOR('',#15682,1.);
#4373=VECTOR('',#15683,1.);
#4374=VECTOR('',#15688,1.);
#4375=VECTOR('',#15689,1.);
#4376=VECTOR('',#15690,1.);
#4377=VECTOR('',#15697,1.);
#4378=VECTOR('',#15698,1.);
#4379=VECTOR('',#15699,1.);
#4380=VECTOR('',#15704,1.);
#4381=VECTOR('',#15705,1.);
#4382=VECTOR('',#15706,1.);
#4383=VECTOR('',#15709,1.);
#4384=VECTOR('',#15710,1.);
#4385=VECTOR('',#15711,1.);
#4386=VECTOR('',#15714,1.);
#4387=VECTOR('',#15715,1.);
#4388=VECTOR('',#15716,1.);
#4389=VECTOR('',#15719,1.);
#4390=VECTOR('',#15720,1.);
#4391=VECTOR('',#15721,1.);
#4392=VECTOR('',#15724,1.);
#4393=VECTOR('',#15725,1.);
#4394=VECTOR('',#15726,1.);
#4395=VECTOR('',#15729,1.);
#4396=VECTOR('',#15730,1.);
#4397=VECTOR('',#15731,1.);
#4398=VECTOR('',#15734,1.);
#4399=VECTOR('',#15735,1.);
#4400=VECTOR('',#15736,1.);
#4401=VECTOR('',#15739,1.);
#4402=VECTOR('',#15740,1.);
#4403=VECTOR('',#15741,1.);
#4404=VECTOR('',#15744,1.);
#4405=VECTOR('',#15745,1.);
#4406=VECTOR('',#15746,1.);
#4407=VECTOR('',#15749,1.);
#4408=VECTOR('',#15750,1.);
#4409=VECTOR('',#15751,1.);
#4410=VECTOR('',#15754,1.);
#4411=VECTOR('',#15755,1.);
#4412=VECTOR('',#15756,1.);
#4413=VECTOR('',#15759,1.);
#4414=VECTOR('',#15760,1.);
#4415=VECTOR('',#15761,1.);
#4416=VECTOR('',#15764,1.);
#4417=VECTOR('',#15765,1.);
#4418=VECTOR('',#15766,1.);
#4419=VECTOR('',#15769,1.);
#4420=VECTOR('',#15770,1.);
#4421=VECTOR('',#15771,1.);
#4422=VECTOR('',#15774,1.);
#4423=VECTOR('',#15775,1.);
#4424=VECTOR('',#15776,1.);
#4425=VECTOR('',#15779,1.);
#4426=VECTOR('',#15780,1.);
#4427=VECTOR('',#15781,1.);
#4428=VECTOR('',#15784,1.);
#4429=VECTOR('',#15785,1.);
#4430=VECTOR('',#15786,1.);
#4431=VECTOR('',#15789,1.);
#4432=VECTOR('',#15790,1.);
#4433=VECTOR('',#15791,1.);
#4434=VECTOR('',#15794,1.);
#4435=VECTOR('',#15795,1.);
#4436=VECTOR('',#15796,1.);
#4437=VECTOR('',#15799,1.);
#4438=VECTOR('',#15800,1.);
#4439=VECTOR('',#15801,1.);
#4440=VECTOR('',#15804,1.);
#4441=VECTOR('',#15805,1.);
#4442=VECTOR('',#15806,1.);
#4443=VECTOR('',#15809,1.);
#4444=VECTOR('',#15810,1.);
#4445=VECTOR('',#15811,1.);
#4446=VECTOR('',#15814,1.);
#4447=VECTOR('',#15815,1.);
#4448=VECTOR('',#15816,1.);
#4449=VECTOR('',#15819,1.);
#4450=VECTOR('',#15820,1.);
#4451=VECTOR('',#15821,1.);
#4452=VECTOR('',#15824,1.);
#4453=VECTOR('',#15825,1.);
#4454=VECTOR('',#15826,1.);
#4455=VECTOR('',#15829,1.);
#4456=VECTOR('',#15830,1.);
#4457=VECTOR('',#15831,1.);
#4458=VECTOR('',#15834,1.);
#4459=VECTOR('',#15835,1.);
#4460=VECTOR('',#15836,1.);
#4461=VECTOR('',#15839,1.);
#4462=VECTOR('',#15840,1.);
#4463=VECTOR('',#15841,1.);
#4464=VECTOR('',#15844,1.);
#4465=VECTOR('',#15845,1.);
#4466=VECTOR('',#15846,1.);
#4467=VECTOR('',#15849,1.);
#4468=VECTOR('',#15850,1.);
#4469=VECTOR('',#15851,1.);
#4470=VECTOR('',#15854,1.);
#4471=VECTOR('',#15855,1.);
#4472=VECTOR('',#15856,1.);
#4473=VECTOR('',#15859,1.);
#4474=VECTOR('',#15860,1.);
#4475=VECTOR('',#15861,1.);
#4476=VECTOR('',#15864,1.);
#4477=VECTOR('',#15865,1.);
#4478=VECTOR('',#15866,1.);
#4479=VECTOR('',#15869,1.);
#4480=VECTOR('',#15870,1.);
#4481=VECTOR('',#15871,1.);
#4482=VECTOR('',#15874,1.);
#4483=VECTOR('',#15875,1.);
#4484=VECTOR('',#15876,1.);
#4485=VECTOR('',#15879,1.);
#4486=VECTOR('',#15880,1.);
#4487=VECTOR('',#15881,1.);
#4488=VECTOR('',#15884,1.);
#4489=VECTOR('',#15885,1.);
#4490=VECTOR('',#15886,1.);
#4491=VECTOR('',#15889,1.);
#4492=VECTOR('',#15890,1.);
#4493=VECTOR('',#15891,1.);
#4494=VECTOR('',#15894,1.);
#4495=VECTOR('',#15895,1.);
#4496=VECTOR('',#15896,1.);
#4497=VECTOR('',#15899,1.);
#4498=VECTOR('',#15900,1.);
#4499=VECTOR('',#15901,1.);
#4500=VECTOR('',#15904,1.);
#4501=VECTOR('',#15905,1.);
#4502=VECTOR('',#15906,1.);
#4503=VECTOR('',#15909,1.);
#4504=VECTOR('',#15910,1.);
#4505=VECTOR('',#15911,1.);
#4506=VECTOR('',#15914,1.);
#4507=VECTOR('',#15915,1.);
#4508=VECTOR('',#15916,1.);
#4509=VECTOR('',#15919,1.);
#4510=VECTOR('',#15920,1.);
#4511=VECTOR('',#15921,1.);
#4512=VECTOR('',#15924,1.);
#4513=VECTOR('',#15925,1.);
#4514=VECTOR('',#15926,1.);
#4515=VECTOR('',#15929,1.);
#4516=VECTOR('',#15930,1.);
#4517=VECTOR('',#15931,1.);
#4518=VECTOR('',#15934,1.);
#4519=VECTOR('',#15935,1.);
#4520=VECTOR('',#15936,1.);
#4521=VECTOR('',#15939,1.);
#4522=VECTOR('',#15940,1.);
#4523=VECTOR('',#15941,1.);
#4524=VECTOR('',#15944,1.);
#4525=VECTOR('',#15945,1.);
#4526=VECTOR('',#15946,1.);
#4527=VECTOR('',#15949,1.);
#4528=VECTOR('',#15950,1.);
#4529=VECTOR('',#15951,1.);
#4530=VECTOR('',#15954,1.);
#4531=VECTOR('',#15955,1.);
#4532=VECTOR('',#15956,1.);
#4533=VECTOR('',#15959,1.);
#4534=VECTOR('',#15960,1.);
#4535=VECTOR('',#15961,1.);
#4536=VECTOR('',#15964,1.);
#4537=VECTOR('',#15965,1.);
#4538=VECTOR('',#15966,1.);
#4539=VECTOR('',#15969,1.);
#4540=VECTOR('',#15970,1.);
#4541=VECTOR('',#15971,1.);
#4542=VECTOR('',#15974,1.);
#4543=VECTOR('',#15975,1.);
#4544=VECTOR('',#15976,1.);
#4545=VECTOR('',#15979,1.);
#4546=VECTOR('',#15980,1.);
#4547=VECTOR('',#15981,1.);
#4548=VECTOR('',#15984,1.);
#4549=VECTOR('',#15985,1.);
#4550=VECTOR('',#15986,1.);
#4551=VECTOR('',#15989,1.);
#4552=VECTOR('',#15990,1.);
#4553=VECTOR('',#15991,1.);
#4554=VECTOR('',#15994,1.);
#4555=VECTOR('',#15995,1.);
#4556=VECTOR('',#15996,1.);
#4557=VECTOR('',#15999,1.);
#4558=VECTOR('',#16000,1.);
#4559=VECTOR('',#16001,1.);
#4560=VECTOR('',#16004,1.);
#4561=VECTOR('',#16005,1.);
#4562=VECTOR('',#16006,1.);
#4563=VECTOR('',#16009,1.);
#4564=VECTOR('',#16010,1.);
#4565=VECTOR('',#16011,1.);
#4566=VECTOR('',#16014,1.);
#4567=VECTOR('',#16015,1.);
#4568=VECTOR('',#16016,1.);
#4569=VECTOR('',#16019,1.);
#4570=VECTOR('',#16020,1.);
#4571=VECTOR('',#16021,1.);
#4572=VECTOR('',#16024,1.);
#4573=VECTOR('',#16025,1.);
#4574=VECTOR('',#16026,1.);
#4575=VECTOR('',#16029,1.);
#4576=VECTOR('',#16030,1.);
#4577=VECTOR('',#16031,1.);
#4578=VECTOR('',#16034,1.);
#4579=VECTOR('',#16035,1.);
#4580=VECTOR('',#16036,1.);
#4581=VECTOR('',#16039,1.);
#4582=VECTOR('',#16040,1.);
#4583=VECTOR('',#16041,1.);
#4584=VECTOR('',#16044,1.);
#4585=VECTOR('',#16045,1.);
#4586=VECTOR('',#16046,1.);
#4587=VECTOR('',#16049,1.);
#4588=VECTOR('',#16050,1.);
#4589=VECTOR('',#16051,1.);
#4590=VECTOR('',#16054,1.);
#4591=VECTOR('',#16055,1.);
#4592=VECTOR('',#16056,1.);
#4593=VECTOR('',#16059,1.);
#4594=VECTOR('',#16060,1.);
#4595=VECTOR('',#16061,1.);
#4596=VECTOR('',#16064,1.);
#4597=VECTOR('',#16065,1.);
#4598=VECTOR('',#16066,1.);
#4599=VECTOR('',#16069,1.);
#4600=VECTOR('',#16070,1.);
#4601=VECTOR('',#16071,1.);
#4602=VECTOR('',#16074,1.);
#4603=VECTOR('',#16075,1.);
#4604=VECTOR('',#16076,1.);
#4605=VECTOR('',#16079,1.);
#4606=VECTOR('',#16080,1.);
#4607=VECTOR('',#16081,1.);
#4608=VECTOR('',#16084,1.);
#4609=VECTOR('',#16085,1.);
#4610=VECTOR('',#16086,1.);
#4611=VECTOR('',#16089,1.);
#4612=VECTOR('',#16090,1.);
#4613=VECTOR('',#16091,1.);
#4614=VECTOR('',#16094,1.);
#4615=VECTOR('',#16095,1.);
#4616=VECTOR('',#16096,1.);
#4617=VECTOR('',#16099,1.);
#4618=VECTOR('',#16100,1.);
#4619=VECTOR('',#16101,1.);
#4620=VECTOR('',#16104,1.);
#4621=VECTOR('',#16105,1.);
#4622=VECTOR('',#16106,1.);
#4623=VECTOR('',#16109,1.);
#4624=VECTOR('',#16110,1.);
#4625=VECTOR('',#16111,1.);
#4626=VECTOR('',#16114,1.);
#4627=VECTOR('',#16115,1.);
#4628=VECTOR('',#16116,1.);
#4629=VECTOR('',#16119,1.);
#4630=VECTOR('',#16120,1.);
#4631=VECTOR('',#16121,1.);
#4632=VECTOR('',#16124,1.);
#4633=VECTOR('',#16125,1.);
#4634=VECTOR('',#16126,1.);
#4635=VECTOR('',#16129,1.);
#4636=VECTOR('',#16130,1.);
#4637=VECTOR('',#16131,1.);
#4638=VECTOR('',#16134,1.);
#4639=VECTOR('',#16135,1.);
#4640=VECTOR('',#16136,1.);
#4641=VECTOR('',#16139,1.);
#4642=VECTOR('',#16140,1.);
#4643=VECTOR('',#16141,1.);
#4644=VECTOR('',#16144,1.);
#4645=VECTOR('',#16145,1.);
#4646=VECTOR('',#16146,1.);
#4647=VECTOR('',#16149,1.);
#4648=VECTOR('',#16150,1.);
#4649=VECTOR('',#16151,1.);
#4650=VECTOR('',#16154,1.);
#4651=VECTOR('',#16155,1.);
#4652=VECTOR('',#16156,1.);
#4653=VECTOR('',#16159,1.);
#4654=VECTOR('',#16160,1.);
#4655=VECTOR('',#16161,1.);
#4656=VECTOR('',#16164,1.);
#4657=VECTOR('',#16165,1.);
#4658=VECTOR('',#16166,1.);
#4659=VECTOR('',#16169,1.);
#4660=VECTOR('',#16170,1.);
#4661=VECTOR('',#16171,1.);
#4662=VECTOR('',#16174,1.);
#4663=VECTOR('',#16175,1.);
#4664=VECTOR('',#16176,1.);
#4665=VECTOR('',#16179,1.);
#4666=VECTOR('',#16180,1.);
#4667=VECTOR('',#16181,1.);
#4668=VECTOR('',#16184,1.);
#4669=VECTOR('',#16185,1.);
#4670=VECTOR('',#16186,1.);
#4671=VECTOR('',#16189,1.);
#4672=VECTOR('',#16190,1.);
#4673=VECTOR('',#16191,1.);
#4674=VECTOR('',#16194,1.);
#4675=VECTOR('',#16195,1.);
#4676=VECTOR('',#16196,1.);
#4677=VECTOR('',#16199,1.);
#4678=VECTOR('',#16200,1.);
#4679=VECTOR('',#16201,1.);
#4680=VECTOR('',#16204,1.);
#4681=VECTOR('',#16205,1.);
#4682=VECTOR('',#16206,1.);
#4683=VECTOR('',#16209,1.);
#4684=VECTOR('',#16210,1.);
#4685=VECTOR('',#16211,1.);
#4686=VECTOR('',#16214,1.);
#4687=VECTOR('',#16215,1.);
#4688=VECTOR('',#16216,1.);
#4689=VECTOR('',#16219,1.);
#4690=VECTOR('',#16220,1.);
#4691=VECTOR('',#16221,1.);
#4692=VECTOR('',#16224,1.);
#4693=VECTOR('',#16225,1.);
#4694=VECTOR('',#16226,1.);
#4695=VECTOR('',#16229,1.);
#4696=VECTOR('',#16230,1.);
#4697=VECTOR('',#16231,1.);
#4698=VECTOR('',#16234,1.);
#4699=VECTOR('',#16235,1.);
#4700=VECTOR('',#16236,1.);
#4701=VECTOR('',#16239,1.);
#4702=VECTOR('',#16240,1.);
#4703=VECTOR('',#16241,1.);
#4704=VECTOR('',#16244,1.);
#4705=VECTOR('',#16245,1.);
#4706=VECTOR('',#16246,1.);
#4707=VECTOR('',#16249,1.);
#4708=VECTOR('',#16250,1.);
#4709=VECTOR('',#16251,1.);
#4710=VECTOR('',#16254,1.);
#4711=VECTOR('',#16255,1.);
#4712=VECTOR('',#16256,1.);
#4713=VECTOR('',#16259,1.);
#4714=VECTOR('',#16260,1.);
#4715=VECTOR('',#16261,1.);
#4716=VECTOR('',#16264,1.);
#4717=VECTOR('',#16265,1.);
#4718=VECTOR('',#16266,1.);
#4719=VECTOR('',#16269,1.);
#4720=VECTOR('',#16270,1.);
#4721=VECTOR('',#16271,1.);
#4722=VECTOR('',#16274,1.);
#4723=VECTOR('',#16275,1.);
#4724=VECTOR('',#16276,1.);
#4725=VECTOR('',#16279,1.);
#4726=VECTOR('',#16280,1.);
#4727=VECTOR('',#16281,1.);
#4728=VECTOR('',#16284,1.);
#4729=VECTOR('',#16285,1.);
#4730=VECTOR('',#16286,1.);
#4731=VECTOR('',#16289,1.);
#4732=VECTOR('',#16290,1.);
#4733=VECTOR('',#16291,1.);
#4734=VECTOR('',#16294,1.);
#4735=VECTOR('',#16295,1.);
#4736=VECTOR('',#16296,1.);
#4737=VECTOR('',#16299,1.);
#4738=VECTOR('',#16300,1.);
#4739=VECTOR('',#16301,1.);
#4740=VECTOR('',#16304,1.);
#4741=VECTOR('',#16305,1.);
#4742=VECTOR('',#16306,1.);
#4743=VECTOR('',#16309,1.);
#4744=VECTOR('',#16310,1.);
#4745=VECTOR('',#16311,1.);
#4746=VECTOR('',#16314,1.);
#4747=VECTOR('',#16315,1.);
#4748=VECTOR('',#16316,1.);
#4749=VECTOR('',#16319,1.);
#4750=VECTOR('',#16320,1.);
#4751=VECTOR('',#16321,1.);
#4752=VECTOR('',#16324,1.);
#4753=VECTOR('',#16325,1.);
#4754=VECTOR('',#16326,1.);
#4755=VECTOR('',#16329,1.);
#4756=VECTOR('',#16330,1.);
#4757=VECTOR('',#16331,1.);
#4758=VECTOR('',#16334,1.);
#4759=VECTOR('',#16335,1.);
#4760=VECTOR('',#16336,1.);
#4761=VECTOR('',#16339,1.);
#4762=VECTOR('',#16340,1.);
#4763=VECTOR('',#16341,1.);
#4764=VECTOR('',#16344,1.);
#4765=VECTOR('',#16345,1.);
#4766=VECTOR('',#16346,1.);
#4767=VECTOR('',#16349,1.);
#4768=VECTOR('',#16350,1.);
#4769=VECTOR('',#16351,1.);
#4770=VECTOR('',#16354,1.);
#4771=VECTOR('',#16355,1.);
#4772=VECTOR('',#16356,1.);
#4773=VECTOR('',#16359,1.);
#4774=VECTOR('',#16360,1.);
#4775=VECTOR('',#16361,1.);
#4776=VECTOR('',#16364,1.);
#4777=VECTOR('',#16365,1.);
#4778=VECTOR('',#16366,1.);
#4779=VECTOR('',#16369,1.);
#4780=VECTOR('',#16370,1.);
#4781=VECTOR('',#16371,1.);
#4782=VECTOR('',#16374,1.);
#4783=VECTOR('',#16375,1.);
#4784=VECTOR('',#16376,1.);
#4785=VECTOR('',#16379,1.);
#4786=VECTOR('',#16380,1.);
#4787=VECTOR('',#16381,1.);
#4788=VECTOR('',#16384,1.);
#4789=VECTOR('',#16385,1.);
#4790=VECTOR('',#16386,1.);
#4791=VECTOR('',#16389,1.);
#4792=VECTOR('',#16390,1.);
#4793=VECTOR('',#16391,1.);
#4794=VECTOR('',#16394,1.);
#4795=VECTOR('',#16395,1.);
#4796=VECTOR('',#16396,1.);
#4797=VECTOR('',#16399,1.);
#4798=VECTOR('',#16400,1.);
#4799=VECTOR('',#16401,1.);
#4800=VECTOR('',#16404,1.);
#4801=VECTOR('',#16405,1.);
#4802=VECTOR('',#16406,1.);
#4803=VECTOR('',#16409,1.);
#4804=VECTOR('',#16410,1.);
#4805=VECTOR('',#16411,1.);
#4806=VECTOR('',#16414,1.);
#4807=VECTOR('',#16415,1.);
#4808=VECTOR('',#16416,1.);
#4809=VECTOR('',#16419,1.);
#4810=VECTOR('',#16420,1.);
#4811=VECTOR('',#16421,1.);
#4812=VECTOR('',#16424,1.);
#4813=VECTOR('',#16425,1.);
#4814=VECTOR('',#16426,1.);
#4815=VECTOR('',#16429,1.);
#4816=VECTOR('',#16430,1.);
#4817=VECTOR('',#16431,1.);
#4818=VECTOR('',#16434,1.);
#4819=VECTOR('',#16435,1.);
#4820=VECTOR('',#16436,1.);
#4821=VECTOR('',#16439,1.);
#4822=VECTOR('',#16440,1.);
#4823=VECTOR('',#16441,1.);
#4824=VECTOR('',#16444,1.);
#4825=VECTOR('',#16445,1.);
#4826=VECTOR('',#16446,1.);
#4827=VECTOR('',#16449,1.);
#4828=VECTOR('',#16450,1.);
#4829=VECTOR('',#16451,1.);
#4830=VECTOR('',#16454,1.);
#4831=VECTOR('',#16455,1.);
#4832=VECTOR('',#16456,1.);
#4833=VECTOR('',#16459,1.);
#4834=VECTOR('',#16460,1.);
#4835=VECTOR('',#16461,1.);
#4836=VECTOR('',#16464,1.);
#4837=VECTOR('',#16465,1.);
#4838=VECTOR('',#16466,1.);
#4839=VECTOR('',#16469,1.);
#4840=VECTOR('',#16470,1.);
#4841=VECTOR('',#16471,1.);
#4842=VECTOR('',#16474,1.);
#4843=VECTOR('',#16475,1.);
#4844=VECTOR('',#16476,1.);
#4845=VECTOR('',#16479,1.);
#4846=VECTOR('',#16480,1.);
#4847=VECTOR('',#16481,1.);
#4848=VECTOR('',#16484,1.);
#4849=VECTOR('',#16485,1.);
#4850=VECTOR('',#16486,1.);
#4851=VECTOR('',#16489,1.);
#4852=VECTOR('',#16490,1.);
#4853=VECTOR('',#16491,1.);
#4854=VECTOR('',#16494,1.);
#4855=VECTOR('',#16495,1.);
#4856=VECTOR('',#16496,1.);
#4857=VECTOR('',#16499,1.);
#4858=VECTOR('',#16500,1.);
#4859=VECTOR('',#16501,1.);
#4860=VECTOR('',#16504,1.);
#4861=VECTOR('',#16505,1.);
#4862=VECTOR('',#16514,1.);
#4863=VECTOR('',#16515,1.);
#5420=CIRCLE('',#13569,0.425);
#5421=CIRCLE('',#13570,0.425);
#5422=CIRCLE('',#13575,1.);
#5423=CIRCLE('',#13576,1.);
#5424=CIRCLE('',#13578,1.);
#5425=CIRCLE('',#13579,1.);
#5426=CIRCLE('',#13744,1.);
#5427=CIRCLE('',#13745,1.);
#5987=VERTEX_POINT('',#19317);
#5988=VERTEX_POINT('',#19319);
#5989=VERTEX_POINT('',#19324);
#5990=VERTEX_POINT('',#19325);
#5991=VERTEX_POINT('',#19327);
#5992=VERTEX_POINT('',#19329);
#5993=VERTEX_POINT('',#19333);
#5994=VERTEX_POINT('',#19334);
#5995=VERTEX_POINT('',#19336);
#5996=VERTEX_POINT('',#19338);
#5997=VERTEX_POINT('',#19342);
#5998=VERTEX_POINT('',#19344);
#5999=VERTEX_POINT('',#19346);
#6000=VERTEX_POINT('',#19351);
#6001=VERTEX_POINT('',#19353);
#6002=VERTEX_POINT('',#19355);
#6003=VERTEX_POINT('',#19360);
#6004=VERTEX_POINT('',#19362);
#6005=VERTEX_POINT('',#19366);
#6006=VERTEX_POINT('',#19368);
#6007=VERTEX_POINT('',#19372);
#6008=VERTEX_POINT('',#19374);
#6009=VERTEX_POINT('',#19378);
#6010=VERTEX_POINT('',#19380);
#6011=VERTEX_POINT('',#19384);
#6012=VERTEX_POINT('',#19386);
#6013=VERTEX_POINT('',#19390);
#6014=VERTEX_POINT('',#19392);
#6015=VERTEX_POINT('',#19396);
#6016=VERTEX_POINT('',#19398);
#6017=VERTEX_POINT('',#19402);
#6018=VERTEX_POINT('',#19404);
#6019=VERTEX_POINT('',#19408);
#6020=VERTEX_POINT('',#19410);
#6021=VERTEX_POINT('',#19414);
#6022=VERTEX_POINT('',#19416);
#6023=VERTEX_POINT('',#19420);
#6024=VERTEX_POINT('',#19422);
#6025=VERTEX_POINT('',#19426);
#6026=VERTEX_POINT('',#19428);
#6027=VERTEX_POINT('',#19432);
#6028=VERTEX_POINT('',#19434);
#6029=VERTEX_POINT('',#19438);
#6030=VERTEX_POINT('',#19440);
#6031=VERTEX_POINT('',#19444);
#6032=VERTEX_POINT('',#19446);
#6033=VERTEX_POINT('',#19450);
#6034=VERTEX_POINT('',#19452);
#6035=VERTEX_POINT('',#19456);
#6036=VERTEX_POINT('',#19458);
#6037=VERTEX_POINT('',#19462);
#6038=VERTEX_POINT('',#19464);
#6039=VERTEX_POINT('',#19468);
#6040=VERTEX_POINT('',#19470);
#6041=VERTEX_POINT('',#19474);
#6042=VERTEX_POINT('',#19476);
#6043=VERTEX_POINT('',#19480);
#6044=VERTEX_POINT('',#19482);
#6045=VERTEX_POINT('',#19486);
#6046=VERTEX_POINT('',#19488);
#6047=VERTEX_POINT('',#19492);
#6048=VERTEX_POINT('',#19494);
#6049=VERTEX_POINT('',#19498);
#6050=VERTEX_POINT('',#19500);
#6051=VERTEX_POINT('',#19504);
#6052=VERTEX_POINT('',#19506);
#6053=VERTEX_POINT('',#19510);
#6054=VERTEX_POINT('',#19512);
#6055=VERTEX_POINT('',#19516);
#6056=VERTEX_POINT('',#19518);
#6057=VERTEX_POINT('',#19522);
#6058=VERTEX_POINT('',#19524);
#6059=VERTEX_POINT('',#19528);
#6060=VERTEX_POINT('',#19530);
#6061=VERTEX_POINT('',#19534);
#6062=VERTEX_POINT('',#19536);
#6063=VERTEX_POINT('',#19540);
#6064=VERTEX_POINT('',#19542);
#6065=VERTEX_POINT('',#19546);
#6066=VERTEX_POINT('',#19548);
#6067=VERTEX_POINT('',#19552);
#6068=VERTEX_POINT('',#19554);
#6069=VERTEX_POINT('',#19558);
#6070=VERTEX_POINT('',#19560);
#6071=VERTEX_POINT('',#19564);
#6072=VERTEX_POINT('',#19566);
#6073=VERTEX_POINT('',#19570);
#6074=VERTEX_POINT('',#19572);
#6075=VERTEX_POINT('',#19576);
#6076=VERTEX_POINT('',#19578);
#6077=VERTEX_POINT('',#19582);
#6078=VERTEX_POINT('',#19584);
#6079=VERTEX_POINT('',#19588);
#6080=VERTEX_POINT('',#19590);
#6081=VERTEX_POINT('',#19594);
#6082=VERTEX_POINT('',#19596);
#6083=VERTEX_POINT('',#19600);
#6084=VERTEX_POINT('',#19602);
#6085=VERTEX_POINT('',#19606);
#6086=VERTEX_POINT('',#19608);
#6087=VERTEX_POINT('',#19612);
#6088=VERTEX_POINT('',#19614);
#6089=VERTEX_POINT('',#19618);
#6090=VERTEX_POINT('',#19620);
#6091=VERTEX_POINT('',#19624);
#6092=VERTEX_POINT('',#19626);
#6093=VERTEX_POINT('',#19630);
#6094=VERTEX_POINT('',#19632);
#6095=VERTEX_POINT('',#19636);
#6096=VERTEX_POINT('',#19638);
#6097=VERTEX_POINT('',#19642);
#6098=VERTEX_POINT('',#19644);
#6099=VERTEX_POINT('',#19648);
#6100=VERTEX_POINT('',#19650);
#6101=VERTEX_POINT('',#19654);
#6102=VERTEX_POINT('',#19656);
#6103=VERTEX_POINT('',#19660);
#6104=VERTEX_POINT('',#19662);
#6105=VERTEX_POINT('',#19666);
#6106=VERTEX_POINT('',#19668);
#6107=VERTEX_POINT('',#19672);
#6108=VERTEX_POINT('',#19674);
#6109=VERTEX_POINT('',#19678);
#6110=VERTEX_POINT('',#19680);
#6111=VERTEX_POINT('',#19684);
#6112=VERTEX_POINT('',#19686);
#6113=VERTEX_POINT('',#19690);
#6114=VERTEX_POINT('',#19692);
#6115=VERTEX_POINT('',#19696);
#6116=VERTEX_POINT('',#19698);
#6117=VERTEX_POINT('',#19702);
#6118=VERTEX_POINT('',#19704);
#6119=VERTEX_POINT('',#19708);
#6120=VERTEX_POINT('',#19710);
#6121=VERTEX_POINT('',#19714);
#6122=VERTEX_POINT('',#19716);
#6123=VERTEX_POINT('',#19720);
#6124=VERTEX_POINT('',#19722);
#6125=VERTEX_POINT('',#19726);
#6126=VERTEX_POINT('',#19728);
#6127=VERTEX_POINT('',#19732);
#6128=VERTEX_POINT('',#19734);
#6129=VERTEX_POINT('',#19738);
#6130=VERTEX_POINT('',#19740);
#6131=VERTEX_POINT('',#19744);
#6132=VERTEX_POINT('',#19746);
#6133=VERTEX_POINT('',#19750);
#6134=VERTEX_POINT('',#19752);
#6135=VERTEX_POINT('',#19756);
#6136=VERTEX_POINT('',#19758);
#6137=VERTEX_POINT('',#19762);
#6138=VERTEX_POINT('',#19764);
#6139=VERTEX_POINT('',#19768);
#6140=VERTEX_POINT('',#19770);
#6141=VERTEX_POINT('',#19774);
#6142=VERTEX_POINT('',#19776);
#6143=VERTEX_POINT('',#19780);
#6144=VERTEX_POINT('',#19782);
#6145=VERTEX_POINT('',#19786);
#6146=VERTEX_POINT('',#19788);
#6147=VERTEX_POINT('',#19792);
#6148=VERTEX_POINT('',#19794);
#6149=VERTEX_POINT('',#19798);
#6150=VERTEX_POINT('',#19800);
#6151=VERTEX_POINT('',#19804);
#6152=VERTEX_POINT('',#19806);
#6153=VERTEX_POINT('',#19810);
#6154=VERTEX_POINT('',#19812);
#6155=VERTEX_POINT('',#19816);
#6156=VERTEX_POINT('',#19818);
#6157=VERTEX_POINT('',#19822);
#6158=VERTEX_POINT('',#19824);
#6159=VERTEX_POINT('',#19828);
#6160=VERTEX_POINT('',#19830);
#6161=VERTEX_POINT('',#19834);
#6162=VERTEX_POINT('',#19836);
#6163=VERTEX_POINT('',#19840);
#6164=VERTEX_POINT('',#19842);
#6165=VERTEX_POINT('',#19846);
#6166=VERTEX_POINT('',#19848);
#6167=VERTEX_POINT('',#19852);
#6168=VERTEX_POINT('',#19854);
#6169=VERTEX_POINT('',#19858);
#6170=VERTEX_POINT('',#19860);
#6171=VERTEX_POINT('',#19864);
#6172=VERTEX_POINT('',#19866);
#6173=VERTEX_POINT('',#19870);
#6174=VERTEX_POINT('',#19872);
#6175=VERTEX_POINT('',#19876);
#6176=VERTEX_POINT('',#19878);
#6177=VERTEX_POINT('',#19882);
#6178=VERTEX_POINT('',#19884);
#6179=VERTEX_POINT('',#19888);
#6180=VERTEX_POINT('',#19890);
#6181=VERTEX_POINT('',#19894);
#6182=VERTEX_POINT('',#19896);
#6183=VERTEX_POINT('',#19900);
#6184=VERTEX_POINT('',#19902);
#6185=VERTEX_POINT('',#19906);
#6186=VERTEX_POINT('',#19908);
#6187=VERTEX_POINT('',#19912);
#6188=VERTEX_POINT('',#19914);
#6189=VERTEX_POINT('',#19918);
#6190=VERTEX_POINT('',#19920);
#6191=VERTEX_POINT('',#19924);
#6192=VERTEX_POINT('',#19926);
#6193=VERTEX_POINT('',#19930);
#6194=VERTEX_POINT('',#19932);
#6195=VERTEX_POINT('',#19936);
#6196=VERTEX_POINT('',#19938);
#6197=VERTEX_POINT('',#19942);
#6198=VERTEX_POINT('',#19944);
#6199=VERTEX_POINT('',#19948);
#6200=VERTEX_POINT('',#19950);
#6201=VERTEX_POINT('',#19954);
#6202=VERTEX_POINT('',#19956);
#6203=VERTEX_POINT('',#19960);
#6204=VERTEX_POINT('',#19962);
#6205=VERTEX_POINT('',#19966);
#6206=VERTEX_POINT('',#19968);
#6207=VERTEX_POINT('',#19972);
#6208=VERTEX_POINT('',#19974);
#6209=VERTEX_POINT('',#19978);
#6210=VERTEX_POINT('',#19980);
#6211=VERTEX_POINT('',#19984);
#6212=VERTEX_POINT('',#19986);
#6213=VERTEX_POINT('',#19990);
#6214=VERTEX_POINT('',#19992);
#6215=VERTEX_POINT('',#19996);
#6216=VERTEX_POINT('',#19998);
#6217=VERTEX_POINT('',#20002);
#6218=VERTEX_POINT('',#20004);
#6219=VERTEX_POINT('',#20008);
#6220=VERTEX_POINT('',#20010);
#6221=VERTEX_POINT('',#20014);
#6222=VERTEX_POINT('',#20016);
#6223=VERTEX_POINT('',#20020);
#6224=VERTEX_POINT('',#20022);
#6225=VERTEX_POINT('',#20026);
#6226=VERTEX_POINT('',#20028);
#6227=VERTEX_POINT('',#20032);
#6228=VERTEX_POINT('',#20034);
#6229=VERTEX_POINT('',#20038);
#6230=VERTEX_POINT('',#20040);
#6231=VERTEX_POINT('',#20044);
#6232=VERTEX_POINT('',#20046);
#6233=VERTEX_POINT('',#20050);
#6234=VERTEX_POINT('',#20052);
#6235=VERTEX_POINT('',#20056);
#6236=VERTEX_POINT('',#20058);
#6237=VERTEX_POINT('',#20062);
#6238=VERTEX_POINT('',#20064);
#6239=VERTEX_POINT('',#20068);
#6240=VERTEX_POINT('',#20070);
#6241=VERTEX_POINT('',#20074);
#6242=VERTEX_POINT('',#20076);
#6243=VERTEX_POINT('',#20080);
#6244=VERTEX_POINT('',#20082);
#6245=VERTEX_POINT('',#20086);
#6246=VERTEX_POINT('',#20088);
#6247=VERTEX_POINT('',#20092);
#6248=VERTEX_POINT('',#20094);
#6249=VERTEX_POINT('',#20098);
#6250=VERTEX_POINT('',#20100);
#6251=VERTEX_POINT('',#20104);
#6252=VERTEX_POINT('',#20106);
#6253=VERTEX_POINT('',#20110);
#6254=VERTEX_POINT('',#20112);
#6255=VERTEX_POINT('',#20116);
#6256=VERTEX_POINT('',#20118);
#6257=VERTEX_POINT('',#20122);
#6258=VERTEX_POINT('',#20124);
#6259=VERTEX_POINT('',#20128);
#6260=VERTEX_POINT('',#20130);
#6261=VERTEX_POINT('',#20134);
#6262=VERTEX_POINT('',#20136);
#6263=VERTEX_POINT('',#20140);
#6264=VERTEX_POINT('',#20142);
#6265=VERTEX_POINT('',#20146);
#6266=VERTEX_POINT('',#20148);
#6267=VERTEX_POINT('',#20152);
#6268=VERTEX_POINT('',#20154);
#6269=VERTEX_POINT('',#20158);
#6270=VERTEX_POINT('',#20160);
#6271=VERTEX_POINT('',#20164);
#6272=VERTEX_POINT('',#20166);
#6273=VERTEX_POINT('',#20170);
#6274=VERTEX_POINT('',#20172);
#6275=VERTEX_POINT('',#20176);
#6276=VERTEX_POINT('',#20178);
#6277=VERTEX_POINT('',#20182);
#6278=VERTEX_POINT('',#20184);
#6279=VERTEX_POINT('',#20188);
#6280=VERTEX_POINT('',#20190);
#6281=VERTEX_POINT('',#20194);
#6282=VERTEX_POINT('',#20196);
#6283=VERTEX_POINT('',#20200);
#6284=VERTEX_POINT('',#20202);
#6285=VERTEX_POINT('',#20206);
#6286=VERTEX_POINT('',#20208);
#6287=VERTEX_POINT('',#20212);
#6288=VERTEX_POINT('',#20214);
#6289=VERTEX_POINT('',#20218);
#6290=VERTEX_POINT('',#20220);
#6291=VERTEX_POINT('',#20224);
#6292=VERTEX_POINT('',#20226);
#6293=VERTEX_POINT('',#20230);
#6294=VERTEX_POINT('',#20232);
#6295=VERTEX_POINT('',#20236);
#6296=VERTEX_POINT('',#20238);
#6297=VERTEX_POINT('',#20242);
#6298=VERTEX_POINT('',#20244);
#6299=VERTEX_POINT('',#20248);
#6300=VERTEX_POINT('',#20250);
#6301=VERTEX_POINT('',#20254);
#6302=VERTEX_POINT('',#20256);
#6303=VERTEX_POINT('',#20260);
#6304=VERTEX_POINT('',#20262);
#6305=VERTEX_POINT('',#20266);
#6306=VERTEX_POINT('',#20268);
#6307=VERTEX_POINT('',#20272);
#6308=VERTEX_POINT('',#20274);
#6309=VERTEX_POINT('',#20278);
#6310=VERTEX_POINT('',#20280);
#6311=VERTEX_POINT('',#20284);
#6312=VERTEX_POINT('',#20286);
#6313=VERTEX_POINT('',#20290);
#6314=VERTEX_POINT('',#20292);
#6315=VERTEX_POINT('',#20296);
#6316=VERTEX_POINT('',#20298);
#6317=VERTEX_POINT('',#20302);
#6318=VERTEX_POINT('',#20304);
#6319=VERTEX_POINT('',#20308);
#6320=VERTEX_POINT('',#20310);
#6321=VERTEX_POINT('',#20314);
#6322=VERTEX_POINT('',#20316);
#6323=VERTEX_POINT('',#20325);
#6324=VERTEX_POINT('',#20328);
#7303=EDGE_CURVE('',#5987,#5987,#5420,.T.);
#7304=EDGE_CURVE('',#5987,#5988,#3194,.T.);
#7305=EDGE_CURVE('',#5988,#5988,#5421,.T.);
#7306=EDGE_CURVE('',#5989,#5990,#3195,.T.);
#7307=EDGE_CURVE('',#5991,#5989,#3196,.T.);
#7308=EDGE_CURVE('',#5992,#5991,#3197,.T.);
#7309=EDGE_CURVE('',#5992,#5990,#3198,.T.);
#7310=EDGE_CURVE('',#5993,#5994,#3199,.T.);
#7311=EDGE_CURVE('',#5993,#5995,#3200,.T.);
#7312=EDGE_CURVE('',#5996,#5995,#3201,.T.);
#7313=EDGE_CURVE('',#5994,#5996,#3202,.T.);
#7314=EDGE_CURVE('',#5990,#5997,#5422,.T.);
#7315=EDGE_CURVE('',#5998,#5992,#3203,.T.);
#7316=EDGE_CURVE('',#5998,#5999,#3204,.T.);
#7317=EDGE_CURVE('',#5995,#5999,#3205,.T.);
#7318=EDGE_CURVE('',#5997,#5993,#5423,.T.);
#7319=EDGE_CURVE('',#5994,#6000,#5424,.T.);
#7320=EDGE_CURVE('',#6001,#5996,#3206,.T.);
#7321=EDGE_CURVE('',#6002,#6001,#3207,.T.);
#7322=EDGE_CURVE('',#5991,#6002,#3208,.T.);
#7323=EDGE_CURVE('',#6000,#5989,#5425,.T.);
#7324=EDGE_CURVE('',#6002,#6003,#3209,.T.);
#7325=EDGE_CURVE('',#6004,#6001,#3210,.T.);
#7326=EDGE_CURVE('',#6003,#6004,#3211,.T.);
#7327=EDGE_CURVE('',#6003,#6005,#3212,.T.);
#7328=EDGE_CURVE('',#6006,#6004,#3213,.T.);
#7329=EDGE_CURVE('',#6005,#6006,#3214,.T.);
#7330=EDGE_CURVE('',#6005,#6007,#3215,.T.);
#7331=EDGE_CURVE('',#6008,#6006,#3216,.T.);
#7332=EDGE_CURVE('',#6007,#6008,#3217,.T.);
#7333=EDGE_CURVE('',#6007,#6009,#3218,.T.);
#7334=EDGE_CURVE('',#6010,#6008,#3219,.T.);
#7335=EDGE_CURVE('',#6009,#6010,#3220,.T.);
#7336=EDGE_CURVE('',#6009,#6011,#3221,.T.);
#7337=EDGE_CURVE('',#6012,#6010,#3222,.T.);
#7338=EDGE_CURVE('',#6011,#6012,#3223,.T.);
#7339=EDGE_CURVE('',#6011,#6013,#3224,.T.);
#7340=EDGE_CURVE('',#6014,#6012,#3225,.T.);
#7341=EDGE_CURVE('',#6013,#6014,#3226,.T.);
#7342=EDGE_CURVE('',#6013,#6015,#3227,.T.);
#7343=EDGE_CURVE('',#6016,#6014,#3228,.T.);
#7344=EDGE_CURVE('',#6015,#6016,#3229,.T.);
#7345=EDGE_CURVE('',#6015,#6017,#3230,.T.);
#7346=EDGE_CURVE('',#6018,#6016,#3231,.T.);
#7347=EDGE_CURVE('',#6017,#6018,#3232,.T.);
#7348=EDGE_CURVE('',#6017,#6019,#3233,.T.);
#7349=EDGE_CURVE('',#6020,#6018,#3234,.T.);
#7350=EDGE_CURVE('',#6019,#6020,#3235,.T.);
#7351=EDGE_CURVE('',#6019,#6021,#3236,.T.);
#7352=EDGE_CURVE('',#6022,#6020,#3237,.T.);
#7353=EDGE_CURVE('',#6021,#6022,#3238,.T.);
#7354=EDGE_CURVE('',#6021,#6023,#3239,.T.);
#7355=EDGE_CURVE('',#6024,#6022,#3240,.T.);
#7356=EDGE_CURVE('',#6023,#6024,#3241,.T.);
#7357=EDGE_CURVE('',#6023,#6025,#3242,.T.);
#7358=EDGE_CURVE('',#6026,#6024,#3243,.T.);
#7359=EDGE_CURVE('',#6025,#6026,#3244,.T.);
#7360=EDGE_CURVE('',#6025,#6027,#3245,.T.);
#7361=EDGE_CURVE('',#6028,#6026,#3246,.T.);
#7362=EDGE_CURVE('',#6027,#6028,#3247,.T.);
#7363=EDGE_CURVE('',#6027,#6029,#3248,.T.);
#7364=EDGE_CURVE('',#6030,#6028,#3249,.T.);
#7365=EDGE_CURVE('',#6029,#6030,#3250,.T.);
#7366=EDGE_CURVE('',#6029,#6031,#3251,.T.);
#7367=EDGE_CURVE('',#6032,#6030,#3252,.T.);
#7368=EDGE_CURVE('',#6031,#6032,#3253,.T.);
#7369=EDGE_CURVE('',#6031,#6033,#3254,.T.);
#7370=EDGE_CURVE('',#6034,#6032,#3255,.T.);
#7371=EDGE_CURVE('',#6033,#6034,#3256,.T.);
#7372=EDGE_CURVE('',#6033,#6035,#3257,.T.);
#7373=EDGE_CURVE('',#6036,#6034,#3258,.T.);
#7374=EDGE_CURVE('',#6035,#6036,#3259,.T.);
#7375=EDGE_CURVE('',#6035,#6037,#3260,.T.);
#7376=EDGE_CURVE('',#6038,#6036,#3261,.T.);
#7377=EDGE_CURVE('',#6037,#6038,#3262,.T.);
#7378=EDGE_CURVE('',#6037,#6039,#3263,.T.);
#7379=EDGE_CURVE('',#6040,#6038,#3264,.T.);
#7380=EDGE_CURVE('',#6039,#6040,#3265,.T.);
#7381=EDGE_CURVE('',#6039,#6041,#3266,.T.);
#7382=EDGE_CURVE('',#6042,#6040,#3267,.T.);
#7383=EDGE_CURVE('',#6041,#6042,#3268,.T.);
#7384=EDGE_CURVE('',#6041,#6043,#3269,.T.);
#7385=EDGE_CURVE('',#6044,#6042,#3270,.T.);
#7386=EDGE_CURVE('',#6043,#6044,#3271,.T.);
#7387=EDGE_CURVE('',#6043,#6045,#3272,.T.);
#7388=EDGE_CURVE('',#6046,#6044,#3273,.T.);
#7389=EDGE_CURVE('',#6045,#6046,#3274,.T.);
#7390=EDGE_CURVE('',#6045,#6047,#3275,.T.);
#7391=EDGE_CURVE('',#6048,#6046,#3276,.T.);
#7392=EDGE_CURVE('',#6047,#6048,#3277,.T.);
#7393=EDGE_CURVE('',#6047,#6049,#3278,.T.);
#7394=EDGE_CURVE('',#6050,#6048,#3279,.T.);
#7395=EDGE_CURVE('',#6049,#6050,#3280,.T.);
#7396=EDGE_CURVE('',#6049,#6051,#3281,.T.);
#7397=EDGE_CURVE('',#6052,#6050,#3282,.T.);
#7398=EDGE_CURVE('',#6051,#6052,#3283,.T.);
#7399=EDGE_CURVE('',#6051,#6053,#3284,.T.);
#7400=EDGE_CURVE('',#6054,#6052,#3285,.T.);
#7401=EDGE_CURVE('',#6053,#6054,#3286,.T.);
#7402=EDGE_CURVE('',#6053,#6055,#3287,.T.);
#7403=EDGE_CURVE('',#6056,#6054,#3288,.T.);
#7404=EDGE_CURVE('',#6055,#6056,#3289,.T.);
#7405=EDGE_CURVE('',#6055,#6057,#3290,.T.);
#7406=EDGE_CURVE('',#6058,#6056,#3291,.T.);
#7407=EDGE_CURVE('',#6057,#6058,#3292,.T.);
#7408=EDGE_CURVE('',#6057,#6059,#3293,.T.);
#7409=EDGE_CURVE('',#6060,#6058,#3294,.T.);
#7410=EDGE_CURVE('',#6059,#6060,#3295,.T.);
#7411=EDGE_CURVE('',#6059,#6061,#3296,.T.);
#7412=EDGE_CURVE('',#6062,#6060,#3297,.T.);
#7413=EDGE_CURVE('',#6061,#6062,#3298,.T.);
#7414=EDGE_CURVE('',#6061,#6063,#3299,.T.);
#7415=EDGE_CURVE('',#6064,#6062,#3300,.T.);
#7416=EDGE_CURVE('',#6063,#6064,#3301,.T.);
#7417=EDGE_CURVE('',#6063,#6065,#3302,.T.);
#7418=EDGE_CURVE('',#6066,#6064,#3303,.T.);
#7419=EDGE_CURVE('',#6065,#6066,#3304,.T.);
#7420=EDGE_CURVE('',#6065,#6067,#3305,.T.);
#7421=EDGE_CURVE('',#6068,#6066,#3306,.T.);
#7422=EDGE_CURVE('',#6067,#6068,#3307,.T.);
#7423=EDGE_CURVE('',#6067,#6069,#3308,.T.);
#7424=EDGE_CURVE('',#6070,#6068,#3309,.T.);
#7425=EDGE_CURVE('',#6069,#6070,#3310,.T.);
#7426=EDGE_CURVE('',#6069,#6071,#3311,.T.);
#7427=EDGE_CURVE('',#6072,#6070,#3312,.T.);
#7428=EDGE_CURVE('',#6071,#6072,#3313,.T.);
#7429=EDGE_CURVE('',#6071,#6073,#3314,.T.);
#7430=EDGE_CURVE('',#6074,#6072,#3315,.T.);
#7431=EDGE_CURVE('',#6073,#6074,#3316,.T.);
#7432=EDGE_CURVE('',#6073,#6075,#3317,.T.);
#7433=EDGE_CURVE('',#6076,#6074,#3318,.T.);
#7434=EDGE_CURVE('',#6075,#6076,#3319,.T.);
#7435=EDGE_CURVE('',#6075,#6077,#3320,.T.);
#7436=EDGE_CURVE('',#6078,#6076,#3321,.T.);
#7437=EDGE_CURVE('',#6077,#6078,#3322,.T.);
#7438=EDGE_CURVE('',#6077,#6079,#3323,.T.);
#7439=EDGE_CURVE('',#6080,#6078,#3324,.T.);
#7440=EDGE_CURVE('',#6079,#6080,#3325,.T.);
#7441=EDGE_CURVE('',#6079,#6081,#3326,.T.);
#7442=EDGE_CURVE('',#6082,#6080,#3327,.T.);
#7443=EDGE_CURVE('',#6081,#6082,#3328,.T.);
#7444=EDGE_CURVE('',#6081,#6083,#3329,.T.);
#7445=EDGE_CURVE('',#6084,#6082,#3330,.T.);
#7446=EDGE_CURVE('',#6083,#6084,#3331,.T.);
#7447=EDGE_CURVE('',#6083,#6085,#3332,.T.);
#7448=EDGE_CURVE('',#6086,#6084,#3333,.T.);
#7449=EDGE_CURVE('',#6085,#6086,#3334,.T.);
#7450=EDGE_CURVE('',#6085,#6087,#3335,.T.);
#7451=EDGE_CURVE('',#6088,#6086,#3336,.T.);
#7452=EDGE_CURVE('',#6087,#6088,#3337,.T.);
#7453=EDGE_CURVE('',#6087,#6089,#3338,.T.);
#7454=EDGE_CURVE('',#6090,#6088,#3339,.T.);
#7455=EDGE_CURVE('',#6089,#6090,#3340,.T.);
#7456=EDGE_CURVE('',#6089,#6091,#3341,.T.);
#7457=EDGE_CURVE('',#6092,#6090,#3342,.T.);
#7458=EDGE_CURVE('',#6091,#6092,#3343,.T.);
#7459=EDGE_CURVE('',#6091,#6093,#3344,.T.);
#7460=EDGE_CURVE('',#6094,#6092,#3345,.T.);
#7461=EDGE_CURVE('',#6093,#6094,#3346,.T.);
#7462=EDGE_CURVE('',#6093,#6095,#3347,.T.);
#7463=EDGE_CURVE('',#6096,#6094,#3348,.T.);
#7464=EDGE_CURVE('',#6095,#6096,#3349,.T.);
#7465=EDGE_CURVE('',#6095,#6097,#3350,.T.);
#7466=EDGE_CURVE('',#6098,#6096,#3351,.T.);
#7467=EDGE_CURVE('',#6097,#6098,#3352,.T.);
#7468=EDGE_CURVE('',#6097,#6099,#3353,.T.);
#7469=EDGE_CURVE('',#6100,#6098,#3354,.T.);
#7470=EDGE_CURVE('',#6099,#6100,#3355,.T.);
#7471=EDGE_CURVE('',#6099,#6101,#3356,.T.);
#7472=EDGE_CURVE('',#6102,#6100,#3357,.T.);
#7473=EDGE_CURVE('',#6101,#6102,#3358,.T.);
#7474=EDGE_CURVE('',#6101,#6103,#3359,.T.);
#7475=EDGE_CURVE('',#6104,#6102,#3360,.T.);
#7476=EDGE_CURVE('',#6103,#6104,#3361,.T.);
#7477=EDGE_CURVE('',#6103,#6105,#3362,.T.);
#7478=EDGE_CURVE('',#6106,#6104,#3363,.T.);
#7479=EDGE_CURVE('',#6105,#6106,#3364,.T.);
#7480=EDGE_CURVE('',#6105,#6107,#3365,.T.);
#7481=EDGE_CURVE('',#6108,#6106,#3366,.T.);
#7482=EDGE_CURVE('',#6107,#6108,#3367,.T.);
#7483=EDGE_CURVE('',#6107,#6109,#3368,.T.);
#7484=EDGE_CURVE('',#6110,#6108,#3369,.T.);
#7485=EDGE_CURVE('',#6109,#6110,#3370,.T.);
#7486=EDGE_CURVE('',#6109,#6111,#3371,.T.);
#7487=EDGE_CURVE('',#6112,#6110,#3372,.T.);
#7488=EDGE_CURVE('',#6111,#6112,#3373,.T.);
#7489=EDGE_CURVE('',#6111,#6113,#3374,.T.);
#7490=EDGE_CURVE('',#6114,#6112,#3375,.T.);
#7491=EDGE_CURVE('',#6113,#6114,#3376,.T.);
#7492=EDGE_CURVE('',#6113,#6115,#3377,.T.);
#7493=EDGE_CURVE('',#6116,#6114,#3378,.T.);
#7494=EDGE_CURVE('',#6115,#6116,#3379,.T.);
#7495=EDGE_CURVE('',#6115,#6117,#3380,.T.);
#7496=EDGE_CURVE('',#6118,#6116,#3381,.T.);
#7497=EDGE_CURVE('',#6117,#6118,#3382,.T.);
#7498=EDGE_CURVE('',#6117,#6119,#3383,.T.);
#7499=EDGE_CURVE('',#6120,#6118,#3384,.T.);
#7500=EDGE_CURVE('',#6119,#6120,#3385,.T.);
#7501=EDGE_CURVE('',#6119,#6121,#3386,.T.);
#7502=EDGE_CURVE('',#6122,#6120,#3387,.T.);
#7503=EDGE_CURVE('',#6121,#6122,#3388,.T.);
#7504=EDGE_CURVE('',#6121,#6123,#3389,.T.);
#7505=EDGE_CURVE('',#6124,#6122,#3390,.T.);
#7506=EDGE_CURVE('',#6123,#6124,#3391,.T.);
#7507=EDGE_CURVE('',#6123,#6125,#3392,.T.);
#7508=EDGE_CURVE('',#6126,#6124,#3393,.T.);
#7509=EDGE_CURVE('',#6125,#6126,#3394,.T.);
#7510=EDGE_CURVE('',#6125,#6127,#3395,.T.);
#7511=EDGE_CURVE('',#6128,#6126,#3396,.T.);
#7512=EDGE_CURVE('',#6127,#6128,#3397,.T.);
#7513=EDGE_CURVE('',#6127,#6129,#3398,.T.);
#7514=EDGE_CURVE('',#6130,#6128,#3399,.T.);
#7515=EDGE_CURVE('',#6129,#6130,#3400,.T.);
#7516=EDGE_CURVE('',#6129,#6131,#3401,.T.);
#7517=EDGE_CURVE('',#6132,#6130,#3402,.T.);
#7518=EDGE_CURVE('',#6131,#6132,#3403,.T.);
#7519=EDGE_CURVE('',#6131,#6133,#3404,.T.);
#7520=EDGE_CURVE('',#6134,#6132,#3405,.T.);
#7521=EDGE_CURVE('',#6133,#6134,#3406,.T.);
#7522=EDGE_CURVE('',#6133,#6135,#3407,.T.);
#7523=EDGE_CURVE('',#6136,#6134,#3408,.T.);
#7524=EDGE_CURVE('',#6135,#6136,#3409,.T.);
#7525=EDGE_CURVE('',#6135,#6137,#3410,.T.);
#7526=EDGE_CURVE('',#6138,#6136,#3411,.T.);
#7527=EDGE_CURVE('',#6137,#6138,#3412,.T.);
#7528=EDGE_CURVE('',#6137,#6139,#3413,.T.);
#7529=EDGE_CURVE('',#6140,#6138,#3414,.T.);
#7530=EDGE_CURVE('',#6139,#6140,#3415,.T.);
#7531=EDGE_CURVE('',#6139,#6141,#3416,.T.);
#7532=EDGE_CURVE('',#6142,#6140,#3417,.T.);
#7533=EDGE_CURVE('',#6141,#6142,#3418,.T.);
#7534=EDGE_CURVE('',#6141,#6143,#3419,.T.);
#7535=EDGE_CURVE('',#6144,#6142,#3420,.T.);
#7536=EDGE_CURVE('',#6143,#6144,#3421,.T.);
#7537=EDGE_CURVE('',#6143,#6145,#3422,.T.);
#7538=EDGE_CURVE('',#6146,#6144,#3423,.T.);
#7539=EDGE_CURVE('',#6145,#6146,#3424,.T.);
#7540=EDGE_CURVE('',#6145,#6147,#3425,.T.);
#7541=EDGE_CURVE('',#6148,#6146,#3426,.T.);
#7542=EDGE_CURVE('',#6147,#6148,#3427,.T.);
#7543=EDGE_CURVE('',#6147,#6149,#3428,.T.);
#7544=EDGE_CURVE('',#6150,#6148,#3429,.T.);
#7545=EDGE_CURVE('',#6149,#6150,#3430,.T.);
#7546=EDGE_CURVE('',#6149,#6151,#3431,.T.);
#7547=EDGE_CURVE('',#6152,#6150,#3432,.T.);
#7548=EDGE_CURVE('',#6151,#6152,#3433,.T.);
#7549=EDGE_CURVE('',#6151,#6153,#3434,.T.);
#7550=EDGE_CURVE('',#6154,#6152,#3435,.T.);
#7551=EDGE_CURVE('',#6153,#6154,#3436,.T.);
#7552=EDGE_CURVE('',#6153,#6155,#3437,.T.);
#7553=EDGE_CURVE('',#6156,#6154,#3438,.T.);
#7554=EDGE_CURVE('',#6155,#6156,#3439,.T.);
#7555=EDGE_CURVE('',#6155,#6157,#3440,.T.);
#7556=EDGE_CURVE('',#6158,#6156,#3441,.T.);
#7557=EDGE_CURVE('',#6157,#6158,#3442,.T.);
#7558=EDGE_CURVE('',#6157,#6159,#3443,.T.);
#7559=EDGE_CURVE('',#6160,#6158,#3444,.T.);
#7560=EDGE_CURVE('',#6159,#6160,#3445,.T.);
#7561=EDGE_CURVE('',#6159,#6161,#3446,.T.);
#7562=EDGE_CURVE('',#6162,#6160,#3447,.T.);
#7563=EDGE_CURVE('',#6161,#6162,#3448,.T.);
#7564=EDGE_CURVE('',#6161,#6163,#3449,.T.);
#7565=EDGE_CURVE('',#6164,#6162,#3450,.T.);
#7566=EDGE_CURVE('',#6163,#6164,#3451,.T.);
#7567=EDGE_CURVE('',#6163,#6165,#3452,.T.);
#7568=EDGE_CURVE('',#6166,#6164,#3453,.T.);
#7569=EDGE_CURVE('',#6165,#6166,#3454,.T.);
#7570=EDGE_CURVE('',#6165,#6167,#3455,.T.);
#7571=EDGE_CURVE('',#6168,#6166,#3456,.T.);
#7572=EDGE_CURVE('',#6167,#6168,#3457,.T.);
#7573=EDGE_CURVE('',#6167,#6169,#3458,.T.);
#7574=EDGE_CURVE('',#6170,#6168,#3459,.T.);
#7575=EDGE_CURVE('',#6169,#6170,#3460,.T.);
#7576=EDGE_CURVE('',#6169,#6171,#3461,.T.);
#7577=EDGE_CURVE('',#6172,#6170,#3462,.T.);
#7578=EDGE_CURVE('',#6171,#6172,#3463,.T.);
#7579=EDGE_CURVE('',#6171,#6173,#3464,.T.);
#7580=EDGE_CURVE('',#6174,#6172,#3465,.T.);
#7581=EDGE_CURVE('',#6173,#6174,#3466,.T.);
#7582=EDGE_CURVE('',#6173,#6175,#3467,.T.);
#7583=EDGE_CURVE('',#6176,#6174,#3468,.T.);
#7584=EDGE_CURVE('',#6175,#6176,#3469,.T.);
#7585=EDGE_CURVE('',#6175,#6177,#3470,.T.);
#7586=EDGE_CURVE('',#6178,#6176,#3471,.T.);
#7587=EDGE_CURVE('',#6177,#6178,#3472,.T.);
#7588=EDGE_CURVE('',#6177,#6179,#3473,.T.);
#7589=EDGE_CURVE('',#6180,#6178,#3474,.T.);
#7590=EDGE_CURVE('',#6179,#6180,#3475,.T.);
#7591=EDGE_CURVE('',#6179,#6181,#3476,.T.);
#7592=EDGE_CURVE('',#6182,#6180,#3477,.T.);
#7593=EDGE_CURVE('',#6181,#6182,#3478,.T.);
#7594=EDGE_CURVE('',#6181,#6183,#3479,.T.);
#7595=EDGE_CURVE('',#6184,#6182,#3480,.T.);
#7596=EDGE_CURVE('',#6183,#6184,#3481,.T.);
#7597=EDGE_CURVE('',#6183,#6185,#3482,.T.);
#7598=EDGE_CURVE('',#6186,#6184,#3483,.T.);
#7599=EDGE_CURVE('',#6185,#6186,#3484,.T.);
#7600=EDGE_CURVE('',#6185,#6187,#3485,.T.);
#7601=EDGE_CURVE('',#6188,#6186,#3486,.T.);
#7602=EDGE_CURVE('',#6187,#6188,#3487,.T.);
#7603=EDGE_CURVE('',#6187,#6189,#3488,.T.);
#7604=EDGE_CURVE('',#6190,#6188,#3489,.T.);
#7605=EDGE_CURVE('',#6189,#6190,#3490,.T.);
#7606=EDGE_CURVE('',#6189,#6191,#3491,.T.);
#7607=EDGE_CURVE('',#6192,#6190,#3492,.T.);
#7608=EDGE_CURVE('',#6191,#6192,#3493,.T.);
#7609=EDGE_CURVE('',#6191,#6193,#3494,.T.);
#7610=EDGE_CURVE('',#6194,#6192,#3495,.T.);
#7611=EDGE_CURVE('',#6193,#6194,#3496,.T.);
#7612=EDGE_CURVE('',#6193,#6195,#3497,.T.);
#7613=EDGE_CURVE('',#6196,#6194,#3498,.T.);
#7614=EDGE_CURVE('',#6195,#6196,#3499,.T.);
#7615=EDGE_CURVE('',#6195,#6197,#3500,.T.);
#7616=EDGE_CURVE('',#6198,#6196,#3501,.T.);
#7617=EDGE_CURVE('',#6197,#6198,#3502,.T.);
#7618=EDGE_CURVE('',#6197,#6199,#3503,.T.);
#7619=EDGE_CURVE('',#6200,#6198,#3504,.T.);
#7620=EDGE_CURVE('',#6199,#6200,#3505,.T.);
#7621=EDGE_CURVE('',#6199,#6201,#3506,.T.);
#7622=EDGE_CURVE('',#6202,#6200,#3507,.T.);
#7623=EDGE_CURVE('',#6201,#6202,#3508,.T.);
#7624=EDGE_CURVE('',#6201,#6203,#3509,.T.);
#7625=EDGE_CURVE('',#6204,#6202,#3510,.T.);
#7626=EDGE_CURVE('',#6203,#6204,#3511,.T.);
#7627=EDGE_CURVE('',#6203,#6205,#3512,.T.);
#7628=EDGE_CURVE('',#6206,#6204,#3513,.T.);
#7629=EDGE_CURVE('',#6205,#6206,#3514,.T.);
#7630=EDGE_CURVE('',#6205,#6207,#3515,.T.);
#7631=EDGE_CURVE('',#6208,#6206,#3516,.T.);
#7632=EDGE_CURVE('',#6207,#6208,#3517,.T.);
#7633=EDGE_CURVE('',#6207,#6209,#3518,.T.);
#7634=EDGE_CURVE('',#6210,#6208,#3519,.T.);
#7635=EDGE_CURVE('',#6209,#6210,#3520,.T.);
#7636=EDGE_CURVE('',#6209,#6211,#3521,.T.);
#7637=EDGE_CURVE('',#6212,#6210,#3522,.T.);
#7638=EDGE_CURVE('',#6211,#6212,#3523,.T.);
#7639=EDGE_CURVE('',#6211,#6213,#3524,.T.);
#7640=EDGE_CURVE('',#6214,#6212,#3525,.T.);
#7641=EDGE_CURVE('',#6213,#6214,#3526,.T.);
#7642=EDGE_CURVE('',#6213,#6215,#3527,.T.);
#7643=EDGE_CURVE('',#6216,#6214,#3528,.T.);
#7644=EDGE_CURVE('',#6215,#6216,#3529,.T.);
#7645=EDGE_CURVE('',#6215,#6217,#3530,.T.);
#7646=EDGE_CURVE('',#6218,#6216,#3531,.T.);
#7647=EDGE_CURVE('',#6217,#6218,#3532,.T.);
#7648=EDGE_CURVE('',#6217,#6219,#3533,.T.);
#7649=EDGE_CURVE('',#6220,#6218,#3534,.T.);
#7650=EDGE_CURVE('',#6219,#6220,#3535,.T.);
#7651=EDGE_CURVE('',#6219,#6221,#3536,.T.);
#7652=EDGE_CURVE('',#6222,#6220,#3537,.T.);
#7653=EDGE_CURVE('',#6221,#6222,#3538,.T.);
#7654=EDGE_CURVE('',#6221,#6223,#3539,.T.);
#7655=EDGE_CURVE('',#6224,#6222,#3540,.T.);
#7656=EDGE_CURVE('',#6223,#6224,#3541,.T.);
#7657=EDGE_CURVE('',#6223,#6225,#3542,.T.);
#7658=EDGE_CURVE('',#6226,#6224,#3543,.T.);
#7659=EDGE_CURVE('',#6225,#6226,#3544,.T.);
#7660=EDGE_CURVE('',#6225,#6227,#3545,.T.);
#7661=EDGE_CURVE('',#6228,#6226,#3546,.T.);
#7662=EDGE_CURVE('',#6227,#6228,#3547,.T.);
#7663=EDGE_CURVE('',#6227,#6229,#3548,.T.);
#7664=EDGE_CURVE('',#6230,#6228,#3549,.T.);
#7665=EDGE_CURVE('',#6229,#6230,#3550,.T.);
#7666=EDGE_CURVE('',#6229,#6231,#3551,.T.);
#7667=EDGE_CURVE('',#6232,#6230,#3552,.T.);
#7668=EDGE_CURVE('',#6231,#6232,#3553,.T.);
#7669=EDGE_CURVE('',#6231,#6233,#3554,.T.);
#7670=EDGE_CURVE('',#6234,#6232,#3555,.T.);
#7671=EDGE_CURVE('',#6233,#6234,#3556,.T.);
#7672=EDGE_CURVE('',#6233,#6235,#3557,.T.);
#7673=EDGE_CURVE('',#6236,#6234,#3558,.T.);
#7674=EDGE_CURVE('',#6235,#6236,#3559,.T.);
#7675=EDGE_CURVE('',#6235,#6237,#3560,.T.);
#7676=EDGE_CURVE('',#6238,#6236,#3561,.T.);
#7677=EDGE_CURVE('',#6237,#6238,#3562,.T.);
#7678=EDGE_CURVE('',#6237,#6239,#3563,.T.);
#7679=EDGE_CURVE('',#6240,#6238,#3564,.T.);
#7680=EDGE_CURVE('',#6239,#6240,#3565,.T.);
#7681=EDGE_CURVE('',#6239,#6241,#3566,.T.);
#7682=EDGE_CURVE('',#6242,#6240,#3567,.T.);
#7683=EDGE_CURVE('',#6241,#6242,#3568,.T.);
#7684=EDGE_CURVE('',#6241,#6243,#3569,.T.);
#7685=EDGE_CURVE('',#6244,#6242,#3570,.T.);
#7686=EDGE_CURVE('',#6243,#6244,#3571,.T.);
#7687=EDGE_CURVE('',#6243,#6245,#3572,.T.);
#7688=EDGE_CURVE('',#6246,#6244,#3573,.T.);
#7689=EDGE_CURVE('',#6245,#6246,#3574,.T.);
#7690=EDGE_CURVE('',#6245,#6247,#3575,.T.);
#7691=EDGE_CURVE('',#6248,#6246,#3576,.T.);
#7692=EDGE_CURVE('',#6247,#6248,#3577,.T.);
#7693=EDGE_CURVE('',#6247,#6249,#3578,.T.);
#7694=EDGE_CURVE('',#6250,#6248,#3579,.T.);
#7695=EDGE_CURVE('',#6249,#6250,#3580,.T.);
#7696=EDGE_CURVE('',#6249,#6251,#3581,.T.);
#7697=EDGE_CURVE('',#6252,#6250,#3582,.T.);
#7698=EDGE_CURVE('',#6251,#6252,#3583,.T.);
#7699=EDGE_CURVE('',#6251,#6253,#3584,.T.);
#7700=EDGE_CURVE('',#6254,#6252,#3585,.T.);
#7701=EDGE_CURVE('',#6253,#6254,#3586,.T.);
#7702=EDGE_CURVE('',#6253,#6255,#3587,.T.);
#7703=EDGE_CURVE('',#6256,#6254,#3588,.T.);
#7704=EDGE_CURVE('',#6255,#6256,#3589,.T.);
#7705=EDGE_CURVE('',#6255,#6257,#3590,.T.);
#7706=EDGE_CURVE('',#6258,#6256,#3591,.T.);
#7707=EDGE_CURVE('',#6257,#6258,#3592,.T.);
#7708=EDGE_CURVE('',#6257,#6259,#3593,.T.);
#7709=EDGE_CURVE('',#6260,#6258,#3594,.T.);
#7710=EDGE_CURVE('',#6259,#6260,#3595,.T.);
#7711=EDGE_CURVE('',#6259,#6261,#3596,.T.);
#7712=EDGE_CURVE('',#6262,#6260,#3597,.T.);
#7713=EDGE_CURVE('',#6261,#6262,#3598,.T.);
#7714=EDGE_CURVE('',#6261,#6263,#3599,.T.);
#7715=EDGE_CURVE('',#6264,#6262,#3600,.T.);
#7716=EDGE_CURVE('',#6263,#6264,#3601,.T.);
#7717=EDGE_CURVE('',#6263,#6265,#3602,.T.);
#7718=EDGE_CURVE('',#6266,#6264,#3603,.T.);
#7719=EDGE_CURVE('',#6265,#6266,#3604,.T.);
#7720=EDGE_CURVE('',#6265,#6267,#3605,.T.);
#7721=EDGE_CURVE('',#6268,#6266,#3606,.T.);
#7722=EDGE_CURVE('',#6267,#6268,#3607,.T.);
#7723=EDGE_CURVE('',#6267,#6269,#3608,.T.);
#7724=EDGE_CURVE('',#6270,#6268,#3609,.T.);
#7725=EDGE_CURVE('',#6269,#6270,#3610,.T.);
#7726=EDGE_CURVE('',#6269,#6271,#3611,.T.);
#7727=EDGE_CURVE('',#6272,#6270,#3612,.T.);
#7728=EDGE_CURVE('',#6271,#6272,#3613,.T.);
#7729=EDGE_CURVE('',#6271,#6273,#3614,.T.);
#7730=EDGE_CURVE('',#6274,#6272,#3615,.T.);
#7731=EDGE_CURVE('',#6273,#6274,#3616,.T.);
#7732=EDGE_CURVE('',#6273,#6275,#3617,.T.);
#7733=EDGE_CURVE('',#6276,#6274,#3618,.T.);
#7734=EDGE_CURVE('',#6275,#6276,#3619,.T.);
#7735=EDGE_CURVE('',#6275,#6277,#3620,.T.);
#7736=EDGE_CURVE('',#6278,#6276,#3621,.T.);
#7737=EDGE_CURVE('',#6277,#6278,#3622,.T.);
#7738=EDGE_CURVE('',#6277,#6279,#3623,.T.);
#7739=EDGE_CURVE('',#6280,#6278,#3624,.T.);
#7740=EDGE_CURVE('',#6279,#6280,#3625,.T.);
#7741=EDGE_CURVE('',#6279,#6281,#3626,.T.);
#7742=EDGE_CURVE('',#6282,#6280,#3627,.T.);
#7743=EDGE_CURVE('',#6281,#6282,#3628,.T.);
#7744=EDGE_CURVE('',#6281,#6283,#3629,.T.);
#7745=EDGE_CURVE('',#6284,#6282,#3630,.T.);
#7746=EDGE_CURVE('',#6283,#6284,#3631,.T.);
#7747=EDGE_CURVE('',#6283,#6285,#3632,.T.);
#7748=EDGE_CURVE('',#6286,#6284,#3633,.T.);
#7749=EDGE_CURVE('',#6285,#6286,#3634,.T.);
#7750=EDGE_CURVE('',#6285,#6287,#3635,.T.);
#7751=EDGE_CURVE('',#6288,#6286,#3636,.T.);
#7752=EDGE_CURVE('',#6287,#6288,#3637,.T.);
#7753=EDGE_CURVE('',#6287,#6289,#3638,.T.);
#7754=EDGE_CURVE('',#6290,#6288,#3639,.T.);
#7755=EDGE_CURVE('',#6289,#6290,#3640,.T.);
#7756=EDGE_CURVE('',#6289,#6291,#3641,.T.);
#7757=EDGE_CURVE('',#6292,#6290,#3642,.T.);
#7758=EDGE_CURVE('',#6291,#6292,#3643,.T.);
#7759=EDGE_CURVE('',#6291,#6293,#3644,.T.);
#7760=EDGE_CURVE('',#6294,#6292,#3645,.T.);
#7761=EDGE_CURVE('',#6293,#6294,#3646,.T.);
#7762=EDGE_CURVE('',#6293,#6295,#3647,.T.);
#7763=EDGE_CURVE('',#6296,#6294,#3648,.T.);
#7764=EDGE_CURVE('',#6295,#6296,#3649,.T.);
#7765=EDGE_CURVE('',#6295,#6297,#3650,.T.);
#7766=EDGE_CURVE('',#6298,#6296,#3651,.T.);
#7767=EDGE_CURVE('',#6297,#6298,#3652,.T.);
#7768=EDGE_CURVE('',#6297,#6299,#3653,.T.);
#7769=EDGE_CURVE('',#6300,#6298,#3654,.T.);
#7770=EDGE_CURVE('',#6299,#6300,#3655,.T.);
#7771=EDGE_CURVE('',#6299,#6301,#3656,.T.);
#7772=EDGE_CURVE('',#6302,#6300,#3657,.T.);
#7773=EDGE_CURVE('',#6301,#6302,#3658,.T.);
#7774=EDGE_CURVE('',#6301,#6303,#3659,.T.);
#7775=EDGE_CURVE('',#6304,#6302,#3660,.T.);
#7776=EDGE_CURVE('',#6303,#6304,#3661,.T.);
#7777=EDGE_CURVE('',#6303,#6305,#3662,.T.);
#7778=EDGE_CURVE('',#6306,#6304,#3663,.T.);
#7779=EDGE_CURVE('',#6305,#6306,#3664,.T.);
#7780=EDGE_CURVE('',#6305,#6307,#3665,.T.);
#7781=EDGE_CURVE('',#6308,#6306,#3666,.T.);
#7782=EDGE_CURVE('',#6307,#6308,#3667,.T.);
#7783=EDGE_CURVE('',#6307,#6309,#3668,.T.);
#7784=EDGE_CURVE('',#6310,#6308,#3669,.T.);
#7785=EDGE_CURVE('',#6309,#6310,#3670,.T.);
#7786=EDGE_CURVE('',#6309,#6311,#3671,.T.);
#7787=EDGE_CURVE('',#6312,#6310,#3672,.T.);
#7788=EDGE_CURVE('',#6311,#6312,#3673,.T.);
#7789=EDGE_CURVE('',#6311,#6313,#3674,.T.);
#7790=EDGE_CURVE('',#6314,#6312,#3675,.T.);
#7791=EDGE_CURVE('',#6313,#6314,#3676,.T.);
#7792=EDGE_CURVE('',#6313,#6315,#3677,.T.);
#7793=EDGE_CURVE('',#6316,#6314,#3678,.T.);
#7794=EDGE_CURVE('',#6315,#6316,#3679,.T.);
#7795=EDGE_CURVE('',#6315,#6317,#3680,.T.);
#7796=EDGE_CURVE('',#6318,#6316,#3681,.T.);
#7797=EDGE_CURVE('',#6317,#6318,#3682,.T.);
#7798=EDGE_CURVE('',#6317,#6319,#3683,.T.);
#7799=EDGE_CURVE('',#6320,#6318,#3684,.T.);
#7800=EDGE_CURVE('',#6319,#6320,#3685,.T.);
#7801=EDGE_CURVE('',#6319,#6321,#3686,.T.);
#7802=EDGE_CURVE('',#6322,#6320,#3687,.T.);
#7803=EDGE_CURVE('',#6321,#6322,#3688,.T.);
#7804=EDGE_CURVE('',#6321,#5998,#3689,.T.);
#7805=EDGE_CURVE('',#5999,#6322,#3690,.T.);
#7806=EDGE_CURVE('',#6323,#6323,#5426,.T.);
#7807=EDGE_CURVE('',#6323,#6000,#3691,.T.);
#7808=EDGE_CURVE('',#5997,#6324,#3692,.T.);
#7809=EDGE_CURVE('',#6324,#6324,#5427,.T.);
#9600=ORIENTED_EDGE('',*,*,#7303,.F.);
#9601=ORIENTED_EDGE('',*,*,#7304,.T.);
#9602=ORIENTED_EDGE('',*,*,#7305,.T.);
#9603=ORIENTED_EDGE('',*,*,#7304,.F.);
#9604=ORIENTED_EDGE('',*,*,#7305,.F.);
#9605=ORIENTED_EDGE('',*,*,#7306,.F.);
#9606=ORIENTED_EDGE('',*,*,#7307,.F.);
#9607=ORIENTED_EDGE('',*,*,#7308,.F.);
#9608=ORIENTED_EDGE('',*,*,#7309,.T.);
#9609=ORIENTED_EDGE('',*,*,#7310,.F.);
#9610=ORIENTED_EDGE('',*,*,#7311,.T.);
#9611=ORIENTED_EDGE('',*,*,#7312,.F.);
#9612=ORIENTED_EDGE('',*,*,#7313,.F.);
#9613=ORIENTED_EDGE('',*,*,#7314,.F.);
#9614=ORIENTED_EDGE('',*,*,#7309,.F.);
#9615=ORIENTED_EDGE('',*,*,#7315,.F.);
#9616=ORIENTED_EDGE('',*,*,#7316,.T.);
#9617=ORIENTED_EDGE('',*,*,#7317,.F.);
#9618=ORIENTED_EDGE('',*,*,#7311,.F.);
#9619=ORIENTED_EDGE('',*,*,#7318,.F.);
#9620=ORIENTED_EDGE('',*,*,#7319,.F.);
#9621=ORIENTED_EDGE('',*,*,#7313,.T.);
#9622=ORIENTED_EDGE('',*,*,#7320,.F.);
#9623=ORIENTED_EDGE('',*,*,#7321,.F.);
#9624=ORIENTED_EDGE('',*,*,#7322,.F.);
#9625=ORIENTED_EDGE('',*,*,#7307,.T.);
#9626=ORIENTED_EDGE('',*,*,#7323,.F.);
#9627=ORIENTED_EDGE('',*,*,#7324,.F.);
#9628=ORIENTED_EDGE('',*,*,#7321,.T.);
#9629=ORIENTED_EDGE('',*,*,#7325,.F.);
#9630=ORIENTED_EDGE('',*,*,#7326,.F.);
#9631=ORIENTED_EDGE('',*,*,#7327,.F.);
#9632=ORIENTED_EDGE('',*,*,#7326,.T.);
#9633=ORIENTED_EDGE('',*,*,#7328,.F.);
#9634=ORIENTED_EDGE('',*,*,#7329,.F.);
#9635=ORIENTED_EDGE('',*,*,#7330,.F.);
#9636=ORIENTED_EDGE('',*,*,#7329,.T.);
#9637=ORIENTED_EDGE('',*,*,#7331,.F.);
#9638=ORIENTED_EDGE('',*,*,#7332,.F.);
#9639=ORIENTED_EDGE('',*,*,#7333,.F.);
#9640=ORIENTED_EDGE('',*,*,#7332,.T.);
#9641=ORIENTED_EDGE('',*,*,#7334,.F.);
#9642=ORIENTED_EDGE('',*,*,#7335,.F.);
#9643=ORIENTED_EDGE('',*,*,#7336,.F.);
#9644=ORIENTED_EDGE('',*,*,#7335,.T.);
#9645=ORIENTED_EDGE('',*,*,#7337,.F.);
#9646=ORIENTED_EDGE('',*,*,#7338,.F.);
#9647=ORIENTED_EDGE('',*,*,#7339,.F.);
#9648=ORIENTED_EDGE('',*,*,#7338,.T.);
#9649=ORIENTED_EDGE('',*,*,#7340,.F.);
#9650=ORIENTED_EDGE('',*,*,#7341,.F.);
#9651=ORIENTED_EDGE('',*,*,#7342,.F.);
#9652=ORIENTED_EDGE('',*,*,#7341,.T.);
#9653=ORIENTED_EDGE('',*,*,#7343,.F.);
#9654=ORIENTED_EDGE('',*,*,#7344,.F.);
#9655=ORIENTED_EDGE('',*,*,#7345,.F.);
#9656=ORIENTED_EDGE('',*,*,#7344,.T.);
#9657=ORIENTED_EDGE('',*,*,#7346,.F.);
#9658=ORIENTED_EDGE('',*,*,#7347,.F.);
#9659=ORIENTED_EDGE('',*,*,#7348,.F.);
#9660=ORIENTED_EDGE('',*,*,#7347,.T.);
#9661=ORIENTED_EDGE('',*,*,#7349,.F.);
#9662=ORIENTED_EDGE('',*,*,#7350,.F.);
#9663=ORIENTED_EDGE('',*,*,#7351,.F.);
#9664=ORIENTED_EDGE('',*,*,#7350,.T.);
#9665=ORIENTED_EDGE('',*,*,#7352,.F.);
#9666=ORIENTED_EDGE('',*,*,#7353,.F.);
#9667=ORIENTED_EDGE('',*,*,#7354,.F.);
#9668=ORIENTED_EDGE('',*,*,#7353,.T.);
#9669=ORIENTED_EDGE('',*,*,#7355,.F.);
#9670=ORIENTED_EDGE('',*,*,#7356,.F.);
#9671=ORIENTED_EDGE('',*,*,#7357,.F.);
#9672=ORIENTED_EDGE('',*,*,#7356,.T.);
#9673=ORIENTED_EDGE('',*,*,#7358,.F.);
#9674=ORIENTED_EDGE('',*,*,#7359,.F.);
#9675=ORIENTED_EDGE('',*,*,#7360,.F.);
#9676=ORIENTED_EDGE('',*,*,#7359,.T.);
#9677=ORIENTED_EDGE('',*,*,#7361,.F.);
#9678=ORIENTED_EDGE('',*,*,#7362,.F.);
#9679=ORIENTED_EDGE('',*,*,#7363,.F.);
#9680=ORIENTED_EDGE('',*,*,#7362,.T.);
#9681=ORIENTED_EDGE('',*,*,#7364,.F.);
#9682=ORIENTED_EDGE('',*,*,#7365,.F.);
#9683=ORIENTED_EDGE('',*,*,#7366,.F.);
#9684=ORIENTED_EDGE('',*,*,#7365,.T.);
#9685=ORIENTED_EDGE('',*,*,#7367,.F.);
#9686=ORIENTED_EDGE('',*,*,#7368,.F.);
#9687=ORIENTED_EDGE('',*,*,#7369,.F.);
#9688=ORIENTED_EDGE('',*,*,#7368,.T.);
#9689=ORIENTED_EDGE('',*,*,#7370,.F.);
#9690=ORIENTED_EDGE('',*,*,#7371,.F.);
#9691=ORIENTED_EDGE('',*,*,#7372,.F.);
#9692=ORIENTED_EDGE('',*,*,#7371,.T.);
#9693=ORIENTED_EDGE('',*,*,#7373,.F.);
#9694=ORIENTED_EDGE('',*,*,#7374,.F.);
#9695=ORIENTED_EDGE('',*,*,#7375,.F.);
#9696=ORIENTED_EDGE('',*,*,#7374,.T.);
#9697=ORIENTED_EDGE('',*,*,#7376,.F.);
#9698=ORIENTED_EDGE('',*,*,#7377,.F.);
#9699=ORIENTED_EDGE('',*,*,#7378,.F.);
#9700=ORIENTED_EDGE('',*,*,#7377,.T.);
#9701=ORIENTED_EDGE('',*,*,#7379,.F.);
#9702=ORIENTED_EDGE('',*,*,#7380,.F.);
#9703=ORIENTED_EDGE('',*,*,#7381,.F.);
#9704=ORIENTED_EDGE('',*,*,#7380,.T.);
#9705=ORIENTED_EDGE('',*,*,#7382,.F.);
#9706=ORIENTED_EDGE('',*,*,#7383,.F.);
#9707=ORIENTED_EDGE('',*,*,#7384,.F.);
#9708=ORIENTED_EDGE('',*,*,#7383,.T.);
#9709=ORIENTED_EDGE('',*,*,#7385,.F.);
#9710=ORIENTED_EDGE('',*,*,#7386,.F.);
#9711=ORIENTED_EDGE('',*,*,#7387,.F.);
#9712=ORIENTED_EDGE('',*,*,#7386,.T.);
#9713=ORIENTED_EDGE('',*,*,#7388,.F.);
#9714=ORIENTED_EDGE('',*,*,#7389,.F.);
#9715=ORIENTED_EDGE('',*,*,#7390,.F.);
#9716=ORIENTED_EDGE('',*,*,#7389,.T.);
#9717=ORIENTED_EDGE('',*,*,#7391,.F.);
#9718=ORIENTED_EDGE('',*,*,#7392,.F.);
#9719=ORIENTED_EDGE('',*,*,#7393,.F.);
#9720=ORIENTED_EDGE('',*,*,#7392,.T.);
#9721=ORIENTED_EDGE('',*,*,#7394,.F.);
#9722=ORIENTED_EDGE('',*,*,#7395,.F.);
#9723=ORIENTED_EDGE('',*,*,#7396,.F.);
#9724=ORIENTED_EDGE('',*,*,#7395,.T.);
#9725=ORIENTED_EDGE('',*,*,#7397,.F.);
#9726=ORIENTED_EDGE('',*,*,#7398,.F.);
#9727=ORIENTED_EDGE('',*,*,#7399,.F.);
#9728=ORIENTED_EDGE('',*,*,#7398,.T.);
#9729=ORIENTED_EDGE('',*,*,#7400,.F.);
#9730=ORIENTED_EDGE('',*,*,#7401,.F.);
#9731=ORIENTED_EDGE('',*,*,#7402,.F.);
#9732=ORIENTED_EDGE('',*,*,#7401,.T.);
#9733=ORIENTED_EDGE('',*,*,#7403,.F.);
#9734=ORIENTED_EDGE('',*,*,#7404,.F.);
#9735=ORIENTED_EDGE('',*,*,#7405,.F.);
#9736=ORIENTED_EDGE('',*,*,#7404,.T.);
#9737=ORIENTED_EDGE('',*,*,#7406,.F.);
#9738=ORIENTED_EDGE('',*,*,#7407,.F.);
#9739=ORIENTED_EDGE('',*,*,#7408,.F.);
#9740=ORIENTED_EDGE('',*,*,#7407,.T.);
#9741=ORIENTED_EDGE('',*,*,#7409,.F.);
#9742=ORIENTED_EDGE('',*,*,#7410,.F.);
#9743=ORIENTED_EDGE('',*,*,#7411,.F.);
#9744=ORIENTED_EDGE('',*,*,#7410,.T.);
#9745=ORIENTED_EDGE('',*,*,#7412,.F.);
#9746=ORIENTED_EDGE('',*,*,#7413,.F.);
#9747=ORIENTED_EDGE('',*,*,#7414,.F.);
#9748=ORIENTED_EDGE('',*,*,#7413,.T.);
#9749=ORIENTED_EDGE('',*,*,#7415,.F.);
#9750=ORIENTED_EDGE('',*,*,#7416,.F.);
#9751=ORIENTED_EDGE('',*,*,#7417,.F.);
#9752=ORIENTED_EDGE('',*,*,#7416,.T.);
#9753=ORIENTED_EDGE('',*,*,#7418,.F.);
#9754=ORIENTED_EDGE('',*,*,#7419,.F.);
#9755=ORIENTED_EDGE('',*,*,#7420,.F.);
#9756=ORIENTED_EDGE('',*,*,#7419,.T.);
#9757=ORIENTED_EDGE('',*,*,#7421,.F.);
#9758=ORIENTED_EDGE('',*,*,#7422,.F.);
#9759=ORIENTED_EDGE('',*,*,#7423,.F.);
#9760=ORIENTED_EDGE('',*,*,#7422,.T.);
#9761=ORIENTED_EDGE('',*,*,#7424,.F.);
#9762=ORIENTED_EDGE('',*,*,#7425,.F.);
#9763=ORIENTED_EDGE('',*,*,#7426,.F.);
#9764=ORIENTED_EDGE('',*,*,#7425,.T.);
#9765=ORIENTED_EDGE('',*,*,#7427,.F.);
#9766=ORIENTED_EDGE('',*,*,#7428,.F.);
#9767=ORIENTED_EDGE('',*,*,#7429,.F.);
#9768=ORIENTED_EDGE('',*,*,#7428,.T.);
#9769=ORIENTED_EDGE('',*,*,#7430,.F.);
#9770=ORIENTED_EDGE('',*,*,#7431,.F.);
#9771=ORIENTED_EDGE('',*,*,#7432,.F.);
#9772=ORIENTED_EDGE('',*,*,#7431,.T.);
#9773=ORIENTED_EDGE('',*,*,#7433,.F.);
#9774=ORIENTED_EDGE('',*,*,#7434,.F.);
#9775=ORIENTED_EDGE('',*,*,#7435,.F.);
#9776=ORIENTED_EDGE('',*,*,#7434,.T.);
#9777=ORIENTED_EDGE('',*,*,#7436,.F.);
#9778=ORIENTED_EDGE('',*,*,#7437,.F.);
#9779=ORIENTED_EDGE('',*,*,#7438,.F.);
#9780=ORIENTED_EDGE('',*,*,#7437,.T.);
#9781=ORIENTED_EDGE('',*,*,#7439,.F.);
#9782=ORIENTED_EDGE('',*,*,#7440,.F.);
#9783=ORIENTED_EDGE('',*,*,#7441,.F.);
#9784=ORIENTED_EDGE('',*,*,#7440,.T.);
#9785=ORIENTED_EDGE('',*,*,#7442,.F.);
#9786=ORIENTED_EDGE('',*,*,#7443,.F.);
#9787=ORIENTED_EDGE('',*,*,#7444,.F.);
#9788=ORIENTED_EDGE('',*,*,#7443,.T.);
#9789=ORIENTED_EDGE('',*,*,#7445,.F.);
#9790=ORIENTED_EDGE('',*,*,#7446,.F.);
#9791=ORIENTED_EDGE('',*,*,#7447,.F.);
#9792=ORIENTED_EDGE('',*,*,#7446,.T.);
#9793=ORIENTED_EDGE('',*,*,#7448,.F.);
#9794=ORIENTED_EDGE('',*,*,#7449,.F.);
#9795=ORIENTED_EDGE('',*,*,#7450,.F.);
#9796=ORIENTED_EDGE('',*,*,#7449,.T.);
#9797=ORIENTED_EDGE('',*,*,#7451,.F.);
#9798=ORIENTED_EDGE('',*,*,#7452,.F.);
#9799=ORIENTED_EDGE('',*,*,#7453,.F.);
#9800=ORIENTED_EDGE('',*,*,#7452,.T.);
#9801=ORIENTED_EDGE('',*,*,#7454,.F.);
#9802=ORIENTED_EDGE('',*,*,#7455,.F.);
#9803=ORIENTED_EDGE('',*,*,#7456,.F.);
#9804=ORIENTED_EDGE('',*,*,#7455,.T.);
#9805=ORIENTED_EDGE('',*,*,#7457,.F.);
#9806=ORIENTED_EDGE('',*,*,#7458,.F.);
#9807=ORIENTED_EDGE('',*,*,#7459,.F.);
#9808=ORIENTED_EDGE('',*,*,#7458,.T.);
#9809=ORIENTED_EDGE('',*,*,#7460,.F.);
#9810=ORIENTED_EDGE('',*,*,#7461,.F.);
#9811=ORIENTED_EDGE('',*,*,#7462,.F.);
#9812=ORIENTED_EDGE('',*,*,#7461,.T.);
#9813=ORIENTED_EDGE('',*,*,#7463,.F.);
#9814=ORIENTED_EDGE('',*,*,#7464,.F.);
#9815=ORIENTED_EDGE('',*,*,#7465,.F.);
#9816=ORIENTED_EDGE('',*,*,#7464,.T.);
#9817=ORIENTED_EDGE('',*,*,#7466,.F.);
#9818=ORIENTED_EDGE('',*,*,#7467,.F.);
#9819=ORIENTED_EDGE('',*,*,#7468,.F.);
#9820=ORIENTED_EDGE('',*,*,#7467,.T.);
#9821=ORIENTED_EDGE('',*,*,#7469,.F.);
#9822=ORIENTED_EDGE('',*,*,#7470,.F.);
#9823=ORIENTED_EDGE('',*,*,#7471,.F.);
#9824=ORIENTED_EDGE('',*,*,#7470,.T.);
#9825=ORIENTED_EDGE('',*,*,#7472,.F.);
#9826=ORIENTED_EDGE('',*,*,#7473,.F.);
#9827=ORIENTED_EDGE('',*,*,#7474,.F.);
#9828=ORIENTED_EDGE('',*,*,#7473,.T.);
#9829=ORIENTED_EDGE('',*,*,#7475,.F.);
#9830=ORIENTED_EDGE('',*,*,#7476,.F.);
#9831=ORIENTED_EDGE('',*,*,#7477,.F.);
#9832=ORIENTED_EDGE('',*,*,#7476,.T.);
#9833=ORIENTED_EDGE('',*,*,#7478,.F.);
#9834=ORIENTED_EDGE('',*,*,#7479,.F.);
#9835=ORIENTED_EDGE('',*,*,#7480,.F.);
#9836=ORIENTED_EDGE('',*,*,#7479,.T.);
#9837=ORIENTED_EDGE('',*,*,#7481,.F.);
#9838=ORIENTED_EDGE('',*,*,#7482,.F.);
#9839=ORIENTED_EDGE('',*,*,#7483,.F.);
#9840=ORIENTED_EDGE('',*,*,#7482,.T.);
#9841=ORIENTED_EDGE('',*,*,#7484,.F.);
#9842=ORIENTED_EDGE('',*,*,#7485,.F.);
#9843=ORIENTED_EDGE('',*,*,#7486,.F.);
#9844=ORIENTED_EDGE('',*,*,#7485,.T.);
#9845=ORIENTED_EDGE('',*,*,#7487,.F.);
#9846=ORIENTED_EDGE('',*,*,#7488,.F.);
#9847=ORIENTED_EDGE('',*,*,#7489,.F.);
#9848=ORIENTED_EDGE('',*,*,#7488,.T.);
#9849=ORIENTED_EDGE('',*,*,#7490,.F.);
#9850=ORIENTED_EDGE('',*,*,#7491,.F.);
#9851=ORIENTED_EDGE('',*,*,#7492,.F.);
#9852=ORIENTED_EDGE('',*,*,#7491,.T.);
#9853=ORIENTED_EDGE('',*,*,#7493,.F.);
#9854=ORIENTED_EDGE('',*,*,#7494,.F.);
#9855=ORIENTED_EDGE('',*,*,#7495,.F.);
#9856=ORIENTED_EDGE('',*,*,#7494,.T.);
#9857=ORIENTED_EDGE('',*,*,#7496,.F.);
#9858=ORIENTED_EDGE('',*,*,#7497,.F.);
#9859=ORIENTED_EDGE('',*,*,#7498,.F.);
#9860=ORIENTED_EDGE('',*,*,#7497,.T.);
#9861=ORIENTED_EDGE('',*,*,#7499,.F.);
#9862=ORIENTED_EDGE('',*,*,#7500,.F.);
#9863=ORIENTED_EDGE('',*,*,#7501,.F.);
#9864=ORIENTED_EDGE('',*,*,#7500,.T.);
#9865=ORIENTED_EDGE('',*,*,#7502,.F.);
#9866=ORIENTED_EDGE('',*,*,#7503,.F.);
#9867=ORIENTED_EDGE('',*,*,#7504,.F.);
#9868=ORIENTED_EDGE('',*,*,#7503,.T.);
#9869=ORIENTED_EDGE('',*,*,#7505,.F.);
#9870=ORIENTED_EDGE('',*,*,#7506,.F.);
#9871=ORIENTED_EDGE('',*,*,#7507,.F.);
#9872=ORIENTED_EDGE('',*,*,#7506,.T.);
#9873=ORIENTED_EDGE('',*,*,#7508,.F.);
#9874=ORIENTED_EDGE('',*,*,#7509,.F.);
#9875=ORIENTED_EDGE('',*,*,#7510,.F.);
#9876=ORIENTED_EDGE('',*,*,#7509,.T.);
#9877=ORIENTED_EDGE('',*,*,#7511,.F.);
#9878=ORIENTED_EDGE('',*,*,#7512,.F.);
#9879=ORIENTED_EDGE('',*,*,#7513,.F.);
#9880=ORIENTED_EDGE('',*,*,#7512,.T.);
#9881=ORIENTED_EDGE('',*,*,#7514,.F.);
#9882=ORIENTED_EDGE('',*,*,#7515,.F.);
#9883=ORIENTED_EDGE('',*,*,#7516,.F.);
#9884=ORIENTED_EDGE('',*,*,#7515,.T.);
#9885=ORIENTED_EDGE('',*,*,#7517,.F.);
#9886=ORIENTED_EDGE('',*,*,#7518,.F.);
#9887=ORIENTED_EDGE('',*,*,#7519,.F.);
#9888=ORIENTED_EDGE('',*,*,#7518,.T.);
#9889=ORIENTED_EDGE('',*,*,#7520,.F.);
#9890=ORIENTED_EDGE('',*,*,#7521,.F.);
#9891=ORIENTED_EDGE('',*,*,#7522,.F.);
#9892=ORIENTED_EDGE('',*,*,#7521,.T.);
#9893=ORIENTED_EDGE('',*,*,#7523,.F.);
#9894=ORIENTED_EDGE('',*,*,#7524,.F.);
#9895=ORIENTED_EDGE('',*,*,#7525,.F.);
#9896=ORIENTED_EDGE('',*,*,#7524,.T.);
#9897=ORIENTED_EDGE('',*,*,#7526,.F.);
#9898=ORIENTED_EDGE('',*,*,#7527,.F.);
#9899=ORIENTED_EDGE('',*,*,#7528,.F.);
#9900=ORIENTED_EDGE('',*,*,#7527,.T.);
#9901=ORIENTED_EDGE('',*,*,#7529,.F.);
#9902=ORIENTED_EDGE('',*,*,#7530,.F.);
#9903=ORIENTED_EDGE('',*,*,#7531,.F.);
#9904=ORIENTED_EDGE('',*,*,#7530,.T.);
#9905=ORIENTED_EDGE('',*,*,#7532,.F.);
#9906=ORIENTED_EDGE('',*,*,#7533,.F.);
#9907=ORIENTED_EDGE('',*,*,#7534,.F.);
#9908=ORIENTED_EDGE('',*,*,#7533,.T.);
#9909=ORIENTED_EDGE('',*,*,#7535,.F.);
#9910=ORIENTED_EDGE('',*,*,#7536,.F.);
#9911=ORIENTED_EDGE('',*,*,#7537,.F.);
#9912=ORIENTED_EDGE('',*,*,#7536,.T.);
#9913=ORIENTED_EDGE('',*,*,#7538,.F.);
#9914=ORIENTED_EDGE('',*,*,#7539,.F.);
#9915=ORIENTED_EDGE('',*,*,#7540,.F.);
#9916=ORIENTED_EDGE('',*,*,#7539,.T.);
#9917=ORIENTED_EDGE('',*,*,#7541,.F.);
#9918=ORIENTED_EDGE('',*,*,#7542,.F.);
#9919=ORIENTED_EDGE('',*,*,#7543,.F.);
#9920=ORIENTED_EDGE('',*,*,#7542,.T.);
#9921=ORIENTED_EDGE('',*,*,#7544,.F.);
#9922=ORIENTED_EDGE('',*,*,#7545,.F.);
#9923=ORIENTED_EDGE('',*,*,#7546,.F.);
#9924=ORIENTED_EDGE('',*,*,#7545,.T.);
#9925=ORIENTED_EDGE('',*,*,#7547,.F.);
#9926=ORIENTED_EDGE('',*,*,#7548,.F.);
#9927=ORIENTED_EDGE('',*,*,#7549,.F.);
#9928=ORIENTED_EDGE('',*,*,#7548,.T.);
#9929=ORIENTED_EDGE('',*,*,#7550,.F.);
#9930=ORIENTED_EDGE('',*,*,#7551,.F.);
#9931=ORIENTED_EDGE('',*,*,#7552,.F.);
#9932=ORIENTED_EDGE('',*,*,#7551,.T.);
#9933=ORIENTED_EDGE('',*,*,#7553,.F.);
#9934=ORIENTED_EDGE('',*,*,#7554,.F.);
#9935=ORIENTED_EDGE('',*,*,#7555,.F.);
#9936=ORIENTED_EDGE('',*,*,#7554,.T.);
#9937=ORIENTED_EDGE('',*,*,#7556,.F.);
#9938=ORIENTED_EDGE('',*,*,#7557,.F.);
#9939=ORIENTED_EDGE('',*,*,#7558,.F.);
#9940=ORIENTED_EDGE('',*,*,#7557,.T.);
#9941=ORIENTED_EDGE('',*,*,#7559,.F.);
#9942=ORIENTED_EDGE('',*,*,#7560,.F.);
#9943=ORIENTED_EDGE('',*,*,#7561,.F.);
#9944=ORIENTED_EDGE('',*,*,#7560,.T.);
#9945=ORIENTED_EDGE('',*,*,#7562,.F.);
#9946=ORIENTED_EDGE('',*,*,#7563,.F.);
#9947=ORIENTED_EDGE('',*,*,#7564,.F.);
#9948=ORIENTED_EDGE('',*,*,#7563,.T.);
#9949=ORIENTED_EDGE('',*,*,#7565,.F.);
#9950=ORIENTED_EDGE('',*,*,#7566,.F.);
#9951=ORIENTED_EDGE('',*,*,#7567,.F.);
#9952=ORIENTED_EDGE('',*,*,#7566,.T.);
#9953=ORIENTED_EDGE('',*,*,#7568,.F.);
#9954=ORIENTED_EDGE('',*,*,#7569,.F.);
#9955=ORIENTED_EDGE('',*,*,#7570,.F.);
#9956=ORIENTED_EDGE('',*,*,#7569,.T.);
#9957=ORIENTED_EDGE('',*,*,#7571,.F.);
#9958=ORIENTED_EDGE('',*,*,#7572,.F.);
#9959=ORIENTED_EDGE('',*,*,#7573,.F.);
#9960=ORIENTED_EDGE('',*,*,#7572,.T.);
#9961=ORIENTED_EDGE('',*,*,#7574,.F.);
#9962=ORIENTED_EDGE('',*,*,#7575,.F.);
#9963=ORIENTED_EDGE('',*,*,#7576,.F.);
#9964=ORIENTED_EDGE('',*,*,#7575,.T.);
#9965=ORIENTED_EDGE('',*,*,#7577,.F.);
#9966=ORIENTED_EDGE('',*,*,#7578,.F.);
#9967=ORIENTED_EDGE('',*,*,#7579,.F.);
#9968=ORIENTED_EDGE('',*,*,#7578,.T.);
#9969=ORIENTED_EDGE('',*,*,#7580,.F.);
#9970=ORIENTED_EDGE('',*,*,#7581,.F.);
#9971=ORIENTED_EDGE('',*,*,#7582,.F.);
#9972=ORIENTED_EDGE('',*,*,#7581,.T.);
#9973=ORIENTED_EDGE('',*,*,#7583,.F.);
#9974=ORIENTED_EDGE('',*,*,#7584,.F.);
#9975=ORIENTED_EDGE('',*,*,#7585,.F.);
#9976=ORIENTED_EDGE('',*,*,#7584,.T.);
#9977=ORIENTED_EDGE('',*,*,#7586,.F.);
#9978=ORIENTED_EDGE('',*,*,#7587,.F.);
#9979=ORIENTED_EDGE('',*,*,#7588,.F.);
#9980=ORIENTED_EDGE('',*,*,#7587,.T.);
#9981=ORIENTED_EDGE('',*,*,#7589,.F.);
#9982=ORIENTED_EDGE('',*,*,#7590,.F.);
#9983=ORIENTED_EDGE('',*,*,#7591,.F.);
#9984=ORIENTED_EDGE('',*,*,#7590,.T.);
#9985=ORIENTED_EDGE('',*,*,#7592,.F.);
#9986=ORIENTED_EDGE('',*,*,#7593,.F.);
#9987=ORIENTED_EDGE('',*,*,#7594,.F.);
#9988=ORIENTED_EDGE('',*,*,#7593,.T.);
#9989=ORIENTED_EDGE('',*,*,#7595,.F.);
#9990=ORIENTED_EDGE('',*,*,#7596,.F.);
#9991=ORIENTED_EDGE('',*,*,#7597,.F.);
#9992=ORIENTED_EDGE('',*,*,#7596,.T.);
#9993=ORIENTED_EDGE('',*,*,#7598,.F.);
#9994=ORIENTED_EDGE('',*,*,#7599,.F.);
#9995=ORIENTED_EDGE('',*,*,#7600,.F.);
#9996=ORIENTED_EDGE('',*,*,#7599,.T.);
#9997=ORIENTED_EDGE('',*,*,#7601,.F.);
#9998=ORIENTED_EDGE('',*,*,#7602,.F.);
#9999=ORIENTED_EDGE('',*,*,#7603,.F.);
#10000=ORIENTED_EDGE('',*,*,#7602,.T.);
#10001=ORIENTED_EDGE('',*,*,#7604,.F.);
#10002=ORIENTED_EDGE('',*,*,#7605,.F.);
#10003=ORIENTED_EDGE('',*,*,#7606,.F.);
#10004=ORIENTED_EDGE('',*,*,#7605,.T.);
#10005=ORIENTED_EDGE('',*,*,#7607,.F.);
#10006=ORIENTED_EDGE('',*,*,#7608,.F.);
#10007=ORIENTED_EDGE('',*,*,#7609,.F.);
#10008=ORIENTED_EDGE('',*,*,#7608,.T.);
#10009=ORIENTED_EDGE('',*,*,#7610,.F.);
#10010=ORIENTED_EDGE('',*,*,#7611,.F.);
#10011=ORIENTED_EDGE('',*,*,#7612,.F.);
#10012=ORIENTED_EDGE('',*,*,#7611,.T.);
#10013=ORIENTED_EDGE('',*,*,#7613,.F.);
#10014=ORIENTED_EDGE('',*,*,#7614,.F.);
#10015=ORIENTED_EDGE('',*,*,#7615,.F.);
#10016=ORIENTED_EDGE('',*,*,#7614,.T.);
#10017=ORIENTED_EDGE('',*,*,#7616,.F.);
#10018=ORIENTED_EDGE('',*,*,#7617,.F.);
#10019=ORIENTED_EDGE('',*,*,#7618,.F.);
#10020=ORIENTED_EDGE('',*,*,#7617,.T.);
#10021=ORIENTED_EDGE('',*,*,#7619,.F.);
#10022=ORIENTED_EDGE('',*,*,#7620,.F.);
#10023=ORIENTED_EDGE('',*,*,#7621,.F.);
#10024=ORIENTED_EDGE('',*,*,#7620,.T.);
#10025=ORIENTED_EDGE('',*,*,#7622,.F.);
#10026=ORIENTED_EDGE('',*,*,#7623,.F.);
#10027=ORIENTED_EDGE('',*,*,#7624,.F.);
#10028=ORIENTED_EDGE('',*,*,#7623,.T.);
#10029=ORIENTED_EDGE('',*,*,#7625,.F.);
#10030=ORIENTED_EDGE('',*,*,#7626,.F.);
#10031=ORIENTED_EDGE('',*,*,#7627,.F.);
#10032=ORIENTED_EDGE('',*,*,#7626,.T.);
#10033=ORIENTED_EDGE('',*,*,#7628,.F.);
#10034=ORIENTED_EDGE('',*,*,#7629,.F.);
#10035=ORIENTED_EDGE('',*,*,#7630,.F.);
#10036=ORIENTED_EDGE('',*,*,#7629,.T.);
#10037=ORIENTED_EDGE('',*,*,#7631,.F.);
#10038=ORIENTED_EDGE('',*,*,#7632,.F.);
#10039=ORIENTED_EDGE('',*,*,#7633,.F.);
#10040=ORIENTED_EDGE('',*,*,#7632,.T.);
#10041=ORIENTED_EDGE('',*,*,#7634,.F.);
#10042=ORIENTED_EDGE('',*,*,#7635,.F.);
#10043=ORIENTED_EDGE('',*,*,#7636,.F.);
#10044=ORIENTED_EDGE('',*,*,#7635,.T.);
#10045=ORIENTED_EDGE('',*,*,#7637,.F.);
#10046=ORIENTED_EDGE('',*,*,#7638,.F.);
#10047=ORIENTED_EDGE('',*,*,#7639,.F.);
#10048=ORIENTED_EDGE('',*,*,#7638,.T.);
#10049=ORIENTED_EDGE('',*,*,#7640,.F.);
#10050=ORIENTED_EDGE('',*,*,#7641,.F.);
#10051=ORIENTED_EDGE('',*,*,#7642,.F.);
#10052=ORIENTED_EDGE('',*,*,#7641,.T.);
#10053=ORIENTED_EDGE('',*,*,#7643,.F.);
#10054=ORIENTED_EDGE('',*,*,#7644,.F.);
#10055=ORIENTED_EDGE('',*,*,#7645,.F.);
#10056=ORIENTED_EDGE('',*,*,#7644,.T.);
#10057=ORIENTED_EDGE('',*,*,#7646,.F.);
#10058=ORIENTED_EDGE('',*,*,#7647,.F.);
#10059=ORIENTED_EDGE('',*,*,#7648,.F.);
#10060=ORIENTED_EDGE('',*,*,#7647,.T.);
#10061=ORIENTED_EDGE('',*,*,#7649,.F.);
#10062=ORIENTED_EDGE('',*,*,#7650,.F.);
#10063=ORIENTED_EDGE('',*,*,#7651,.F.);
#10064=ORIENTED_EDGE('',*,*,#7650,.T.);
#10065=ORIENTED_EDGE('',*,*,#7652,.F.);
#10066=ORIENTED_EDGE('',*,*,#7653,.F.);
#10067=ORIENTED_EDGE('',*,*,#7654,.F.);
#10068=ORIENTED_EDGE('',*,*,#7653,.T.);
#10069=ORIENTED_EDGE('',*,*,#7655,.F.);
#10070=ORIENTED_EDGE('',*,*,#7656,.F.);
#10071=ORIENTED_EDGE('',*,*,#7657,.F.);
#10072=ORIENTED_EDGE('',*,*,#7656,.T.);
#10073=ORIENTED_EDGE('',*,*,#7658,.F.);
#10074=ORIENTED_EDGE('',*,*,#7659,.F.);
#10075=ORIENTED_EDGE('',*,*,#7660,.F.);
#10076=ORIENTED_EDGE('',*,*,#7659,.T.);
#10077=ORIENTED_EDGE('',*,*,#7661,.F.);
#10078=ORIENTED_EDGE('',*,*,#7662,.F.);
#10079=ORIENTED_EDGE('',*,*,#7663,.F.);
#10080=ORIENTED_EDGE('',*,*,#7662,.T.);
#10081=ORIENTED_EDGE('',*,*,#7664,.F.);
#10082=ORIENTED_EDGE('',*,*,#7665,.F.);
#10083=ORIENTED_EDGE('',*,*,#7666,.F.);
#10084=ORIENTED_EDGE('',*,*,#7665,.T.);
#10085=ORIENTED_EDGE('',*,*,#7667,.F.);
#10086=ORIENTED_EDGE('',*,*,#7668,.F.);
#10087=ORIENTED_EDGE('',*,*,#7669,.F.);
#10088=ORIENTED_EDGE('',*,*,#7668,.T.);
#10089=ORIENTED_EDGE('',*,*,#7670,.F.);
#10090=ORIENTED_EDGE('',*,*,#7671,.F.);
#10091=ORIENTED_EDGE('',*,*,#7672,.F.);
#10092=ORIENTED_EDGE('',*,*,#7671,.T.);
#10093=ORIENTED_EDGE('',*,*,#7673,.F.);
#10094=ORIENTED_EDGE('',*,*,#7674,.F.);
#10095=ORIENTED_EDGE('',*,*,#7675,.F.);
#10096=ORIENTED_EDGE('',*,*,#7674,.T.);
#10097=ORIENTED_EDGE('',*,*,#7676,.F.);
#10098=ORIENTED_EDGE('',*,*,#7677,.F.);
#10099=ORIENTED_EDGE('',*,*,#7678,.F.);
#10100=ORIENTED_EDGE('',*,*,#7677,.T.);
#10101=ORIENTED_EDGE('',*,*,#7679,.F.);
#10102=ORIENTED_EDGE('',*,*,#7680,.F.);
#10103=ORIENTED_EDGE('',*,*,#7681,.F.);
#10104=ORIENTED_EDGE('',*,*,#7680,.T.);
#10105=ORIENTED_EDGE('',*,*,#7682,.F.);
#10106=ORIENTED_EDGE('',*,*,#7683,.F.);
#10107=ORIENTED_EDGE('',*,*,#7684,.F.);
#10108=ORIENTED_EDGE('',*,*,#7683,.T.);
#10109=ORIENTED_EDGE('',*,*,#7685,.F.);
#10110=ORIENTED_EDGE('',*,*,#7686,.F.);
#10111=ORIENTED_EDGE('',*,*,#7687,.F.);
#10112=ORIENTED_EDGE('',*,*,#7686,.T.);
#10113=ORIENTED_EDGE('',*,*,#7688,.F.);
#10114=ORIENTED_EDGE('',*,*,#7689,.F.);
#10115=ORIENTED_EDGE('',*,*,#7690,.F.);
#10116=ORIENTED_EDGE('',*,*,#7689,.T.);
#10117=ORIENTED_EDGE('',*,*,#7691,.F.);
#10118=ORIENTED_EDGE('',*,*,#7692,.F.);
#10119=ORIENTED_EDGE('',*,*,#7693,.F.);
#10120=ORIENTED_EDGE('',*,*,#7692,.T.);
#10121=ORIENTED_EDGE('',*,*,#7694,.F.);
#10122=ORIENTED_EDGE('',*,*,#7695,.F.);
#10123=ORIENTED_EDGE('',*,*,#7696,.F.);
#10124=ORIENTED_EDGE('',*,*,#7695,.T.);
#10125=ORIENTED_EDGE('',*,*,#7697,.F.);
#10126=ORIENTED_EDGE('',*,*,#7698,.F.);
#10127=ORIENTED_EDGE('',*,*,#7699,.F.);
#10128=ORIENTED_EDGE('',*,*,#7698,.T.);
#10129=ORIENTED_EDGE('',*,*,#7700,.F.);
#10130=ORIENTED_EDGE('',*,*,#7701,.F.);
#10131=ORIENTED_EDGE('',*,*,#7702,.F.);
#10132=ORIENTED_EDGE('',*,*,#7701,.T.);
#10133=ORIENTED_EDGE('',*,*,#7703,.F.);
#10134=ORIENTED_EDGE('',*,*,#7704,.F.);
#10135=ORIENTED_EDGE('',*,*,#7705,.F.);
#10136=ORIENTED_EDGE('',*,*,#7704,.T.);
#10137=ORIENTED_EDGE('',*,*,#7706,.F.);
#10138=ORIENTED_EDGE('',*,*,#7707,.F.);
#10139=ORIENTED_EDGE('',*,*,#7708,.F.);
#10140=ORIENTED_EDGE('',*,*,#7707,.T.);
#10141=ORIENTED_EDGE('',*,*,#7709,.F.);
#10142=ORIENTED_EDGE('',*,*,#7710,.F.);
#10143=ORIENTED_EDGE('',*,*,#7711,.F.);
#10144=ORIENTED_EDGE('',*,*,#7710,.T.);
#10145=ORIENTED_EDGE('',*,*,#7712,.F.);
#10146=ORIENTED_EDGE('',*,*,#7713,.F.);
#10147=ORIENTED_EDGE('',*,*,#7714,.F.);
#10148=ORIENTED_EDGE('',*,*,#7713,.T.);
#10149=ORIENTED_EDGE('',*,*,#7715,.F.);
#10150=ORIENTED_EDGE('',*,*,#7716,.F.);
#10151=ORIENTED_EDGE('',*,*,#7717,.F.);
#10152=ORIENTED_EDGE('',*,*,#7716,.T.);
#10153=ORIENTED_EDGE('',*,*,#7718,.F.);
#10154=ORIENTED_EDGE('',*,*,#7719,.F.);
#10155=ORIENTED_EDGE('',*,*,#7720,.F.);
#10156=ORIENTED_EDGE('',*,*,#7719,.T.);
#10157=ORIENTED_EDGE('',*,*,#7721,.F.);
#10158=ORIENTED_EDGE('',*,*,#7722,.F.);
#10159=ORIENTED_EDGE('',*,*,#7723,.F.);
#10160=ORIENTED_EDGE('',*,*,#7722,.T.);
#10161=ORIENTED_EDGE('',*,*,#7724,.F.);
#10162=ORIENTED_EDGE('',*,*,#7725,.F.);
#10163=ORIENTED_EDGE('',*,*,#7726,.F.);
#10164=ORIENTED_EDGE('',*,*,#7725,.T.);
#10165=ORIENTED_EDGE('',*,*,#7727,.F.);
#10166=ORIENTED_EDGE('',*,*,#7728,.F.);
#10167=ORIENTED_EDGE('',*,*,#7729,.F.);
#10168=ORIENTED_EDGE('',*,*,#7728,.T.);
#10169=ORIENTED_EDGE('',*,*,#7730,.F.);
#10170=ORIENTED_EDGE('',*,*,#7731,.F.);
#10171=ORIENTED_EDGE('',*,*,#7732,.F.);
#10172=ORIENTED_EDGE('',*,*,#7731,.T.);
#10173=ORIENTED_EDGE('',*,*,#7733,.F.);
#10174=ORIENTED_EDGE('',*,*,#7734,.F.);
#10175=ORIENTED_EDGE('',*,*,#7735,.F.);
#10176=ORIENTED_EDGE('',*,*,#7734,.T.);
#10177=ORIENTED_EDGE('',*,*,#7736,.F.);
#10178=ORIENTED_EDGE('',*,*,#7737,.F.);
#10179=ORIENTED_EDGE('',*,*,#7738,.F.);
#10180=ORIENTED_EDGE('',*,*,#7737,.T.);
#10181=ORIENTED_EDGE('',*,*,#7739,.F.);
#10182=ORIENTED_EDGE('',*,*,#7740,.F.);
#10183=ORIENTED_EDGE('',*,*,#7741,.F.);
#10184=ORIENTED_EDGE('',*,*,#7740,.T.);
#10185=ORIENTED_EDGE('',*,*,#7742,.F.);
#10186=ORIENTED_EDGE('',*,*,#7743,.F.);
#10187=ORIENTED_EDGE('',*,*,#7744,.F.);
#10188=ORIENTED_EDGE('',*,*,#7743,.T.);
#10189=ORIENTED_EDGE('',*,*,#7745,.F.);
#10190=ORIENTED_EDGE('',*,*,#7746,.F.);
#10191=ORIENTED_EDGE('',*,*,#7747,.F.);
#10192=ORIENTED_EDGE('',*,*,#7746,.T.);
#10193=ORIENTED_EDGE('',*,*,#7748,.F.);
#10194=ORIENTED_EDGE('',*,*,#7749,.F.);
#10195=ORIENTED_EDGE('',*,*,#7750,.F.);
#10196=ORIENTED_EDGE('',*,*,#7749,.T.);
#10197=ORIENTED_EDGE('',*,*,#7751,.F.);
#10198=ORIENTED_EDGE('',*,*,#7752,.F.);
#10199=ORIENTED_EDGE('',*,*,#7753,.F.);
#10200=ORIENTED_EDGE('',*,*,#7752,.T.);
#10201=ORIENTED_EDGE('',*,*,#7754,.F.);
#10202=ORIENTED_EDGE('',*,*,#7755,.F.);
#10203=ORIENTED_EDGE('',*,*,#7756,.F.);
#10204=ORIENTED_EDGE('',*,*,#7755,.T.);
#10205=ORIENTED_EDGE('',*,*,#7757,.F.);
#10206=ORIENTED_EDGE('',*,*,#7758,.F.);
#10207=ORIENTED_EDGE('',*,*,#7759,.F.);
#10208=ORIENTED_EDGE('',*,*,#7758,.T.);
#10209=ORIENTED_EDGE('',*,*,#7760,.F.);
#10210=ORIENTED_EDGE('',*,*,#7761,.F.);
#10211=ORIENTED_EDGE('',*,*,#7762,.F.);
#10212=ORIENTED_EDGE('',*,*,#7761,.T.);
#10213=ORIENTED_EDGE('',*,*,#7763,.F.);
#10214=ORIENTED_EDGE('',*,*,#7764,.F.);
#10215=ORIENTED_EDGE('',*,*,#7765,.F.);
#10216=ORIENTED_EDGE('',*,*,#7764,.T.);
#10217=ORIENTED_EDGE('',*,*,#7766,.F.);
#10218=ORIENTED_EDGE('',*,*,#7767,.F.);
#10219=ORIENTED_EDGE('',*,*,#7768,.F.);
#10220=ORIENTED_EDGE('',*,*,#7767,.T.);
#10221=ORIENTED_EDGE('',*,*,#7769,.F.);
#10222=ORIENTED_EDGE('',*,*,#7770,.F.);
#10223=ORIENTED_EDGE('',*,*,#7771,.F.);
#10224=ORIENTED_EDGE('',*,*,#7770,.T.);
#10225=ORIENTED_EDGE('',*,*,#7772,.F.);
#10226=ORIENTED_EDGE('',*,*,#7773,.F.);
#10227=ORIENTED_EDGE('',*,*,#7774,.F.);
#10228=ORIENTED_EDGE('',*,*,#7773,.T.);
#10229=ORIENTED_EDGE('',*,*,#7775,.F.);
#10230=ORIENTED_EDGE('',*,*,#7776,.F.);
#10231=ORIENTED_EDGE('',*,*,#7777,.F.);
#10232=ORIENTED_EDGE('',*,*,#7776,.T.);
#10233=ORIENTED_EDGE('',*,*,#7778,.F.);
#10234=ORIENTED_EDGE('',*,*,#7779,.F.);
#10235=ORIENTED_EDGE('',*,*,#7780,.F.);
#10236=ORIENTED_EDGE('',*,*,#7779,.T.);
#10237=ORIENTED_EDGE('',*,*,#7781,.F.);
#10238=ORIENTED_EDGE('',*,*,#7782,.F.);
#10239=ORIENTED_EDGE('',*,*,#7783,.F.);
#10240=ORIENTED_EDGE('',*,*,#7782,.T.);
#10241=ORIENTED_EDGE('',*,*,#7784,.F.);
#10242=ORIENTED_EDGE('',*,*,#7785,.F.);
#10243=ORIENTED_EDGE('',*,*,#7786,.F.);
#10244=ORIENTED_EDGE('',*,*,#7785,.T.);
#10245=ORIENTED_EDGE('',*,*,#7787,.F.);
#10246=ORIENTED_EDGE('',*,*,#7788,.F.);
#10247=ORIENTED_EDGE('',*,*,#7789,.F.);
#10248=ORIENTED_EDGE('',*,*,#7788,.T.);
#10249=ORIENTED_EDGE('',*,*,#7790,.F.);
#10250=ORIENTED_EDGE('',*,*,#7791,.F.);
#10251=ORIENTED_EDGE('',*,*,#7792,.F.);
#10252=ORIENTED_EDGE('',*,*,#7791,.T.);
#10253=ORIENTED_EDGE('',*,*,#7793,.F.);
#10254=ORIENTED_EDGE('',*,*,#7794,.F.);
#10255=ORIENTED_EDGE('',*,*,#7795,.F.);
#10256=ORIENTED_EDGE('',*,*,#7794,.T.);
#10257=ORIENTED_EDGE('',*,*,#7796,.F.);
#10258=ORIENTED_EDGE('',*,*,#7797,.F.);
#10259=ORIENTED_EDGE('',*,*,#7798,.F.);
#10260=ORIENTED_EDGE('',*,*,#7797,.T.);
#10261=ORIENTED_EDGE('',*,*,#7799,.F.);
#10262=ORIENTED_EDGE('',*,*,#7800,.F.);
#10263=ORIENTED_EDGE('',*,*,#7801,.F.);
#10264=ORIENTED_EDGE('',*,*,#7800,.T.);
#10265=ORIENTED_EDGE('',*,*,#7802,.F.);
#10266=ORIENTED_EDGE('',*,*,#7803,.F.);
#10267=ORIENTED_EDGE('',*,*,#7804,.F.);
#10268=ORIENTED_EDGE('',*,*,#7803,.T.);
#10269=ORIENTED_EDGE('',*,*,#7805,.F.);
#10270=ORIENTED_EDGE('',*,*,#7316,.F.);
#10271=ORIENTED_EDGE('',*,*,#7805,.T.);
#10272=ORIENTED_EDGE('',*,*,#7802,.T.);
#10273=ORIENTED_EDGE('',*,*,#7799,.T.);
#10274=ORIENTED_EDGE('',*,*,#7796,.T.);
#10275=ORIENTED_EDGE('',*,*,#7793,.T.);
#10276=ORIENTED_EDGE('',*,*,#7790,.T.);
#10277=ORIENTED_EDGE('',*,*,#7787,.T.);
#10278=ORIENTED_EDGE('',*,*,#7784,.T.);
#10279=ORIENTED_EDGE('',*,*,#7781,.T.);
#10280=ORIENTED_EDGE('',*,*,#7778,.T.);
#10281=ORIENTED_EDGE('',*,*,#7775,.T.);
#10282=ORIENTED_EDGE('',*,*,#7772,.T.);
#10283=ORIENTED_EDGE('',*,*,#7769,.T.);
#10284=ORIENTED_EDGE('',*,*,#7766,.T.);
#10285=ORIENTED_EDGE('',*,*,#7763,.T.);
#10286=ORIENTED_EDGE('',*,*,#7760,.T.);
#10287=ORIENTED_EDGE('',*,*,#7757,.T.);
#10288=ORIENTED_EDGE('',*,*,#7754,.T.);
#10289=ORIENTED_EDGE('',*,*,#7751,.T.);
#10290=ORIENTED_EDGE('',*,*,#7748,.T.);
#10291=ORIENTED_EDGE('',*,*,#7745,.T.);
#10292=ORIENTED_EDGE('',*,*,#7742,.T.);
#10293=ORIENTED_EDGE('',*,*,#7739,.T.);
#10294=ORIENTED_EDGE('',*,*,#7736,.T.);
#10295=ORIENTED_EDGE('',*,*,#7733,.T.);
#10296=ORIENTED_EDGE('',*,*,#7730,.T.);
#10297=ORIENTED_EDGE('',*,*,#7727,.T.);
#10298=ORIENTED_EDGE('',*,*,#7724,.T.);
#10299=ORIENTED_EDGE('',*,*,#7721,.T.);
#10300=ORIENTED_EDGE('',*,*,#7718,.T.);
#10301=ORIENTED_EDGE('',*,*,#7715,.T.);
#10302=ORIENTED_EDGE('',*,*,#7712,.T.);
#10303=ORIENTED_EDGE('',*,*,#7709,.T.);
#10304=ORIENTED_EDGE('',*,*,#7706,.T.);
#10305=ORIENTED_EDGE('',*,*,#7703,.T.);
#10306=ORIENTED_EDGE('',*,*,#7700,.T.);
#10307=ORIENTED_EDGE('',*,*,#7697,.T.);
#10308=ORIENTED_EDGE('',*,*,#7694,.T.);
#10309=ORIENTED_EDGE('',*,*,#7691,.T.);
#10310=ORIENTED_EDGE('',*,*,#7688,.T.);
#10311=ORIENTED_EDGE('',*,*,#7685,.T.);
#10312=ORIENTED_EDGE('',*,*,#7682,.T.);
#10313=ORIENTED_EDGE('',*,*,#7679,.T.);
#10314=ORIENTED_EDGE('',*,*,#7676,.T.);
#10315=ORIENTED_EDGE('',*,*,#7673,.T.);
#10316=ORIENTED_EDGE('',*,*,#7670,.T.);
#10317=ORIENTED_EDGE('',*,*,#7667,.T.);
#10318=ORIENTED_EDGE('',*,*,#7664,.T.);
#10319=ORIENTED_EDGE('',*,*,#7661,.T.);
#10320=ORIENTED_EDGE('',*,*,#7658,.T.);
#10321=ORIENTED_EDGE('',*,*,#7655,.T.);
#10322=ORIENTED_EDGE('',*,*,#7652,.T.);
#10323=ORIENTED_EDGE('',*,*,#7649,.T.);
#10324=ORIENTED_EDGE('',*,*,#7646,.T.);
#10325=ORIENTED_EDGE('',*,*,#7643,.T.);
#10326=ORIENTED_EDGE('',*,*,#7640,.T.);
#10327=ORIENTED_EDGE('',*,*,#7637,.T.);
#10328=ORIENTED_EDGE('',*,*,#7634,.T.);
#10329=ORIENTED_EDGE('',*,*,#7631,.T.);
#10330=ORIENTED_EDGE('',*,*,#7628,.T.);
#10331=ORIENTED_EDGE('',*,*,#7625,.T.);
#10332=ORIENTED_EDGE('',*,*,#7622,.T.);
#10333=ORIENTED_EDGE('',*,*,#7619,.T.);
#10334=ORIENTED_EDGE('',*,*,#7616,.T.);
#10335=ORIENTED_EDGE('',*,*,#7613,.T.);
#10336=ORIENTED_EDGE('',*,*,#7610,.T.);
#10337=ORIENTED_EDGE('',*,*,#7607,.T.);
#10338=ORIENTED_EDGE('',*,*,#7604,.T.);
#10339=ORIENTED_EDGE('',*,*,#7601,.T.);
#10340=ORIENTED_EDGE('',*,*,#7598,.T.);
#10341=ORIENTED_EDGE('',*,*,#7595,.T.);
#10342=ORIENTED_EDGE('',*,*,#7592,.T.);
#10343=ORIENTED_EDGE('',*,*,#7589,.T.);
#10344=ORIENTED_EDGE('',*,*,#7586,.T.);
#10345=ORIENTED_EDGE('',*,*,#7583,.T.);
#10346=ORIENTED_EDGE('',*,*,#7580,.T.);
#10347=ORIENTED_EDGE('',*,*,#7577,.T.);
#10348=ORIENTED_EDGE('',*,*,#7574,.T.);
#10349=ORIENTED_EDGE('',*,*,#7571,.T.);
#10350=ORIENTED_EDGE('',*,*,#7568,.T.);
#10351=ORIENTED_EDGE('',*,*,#7565,.T.);
#10352=ORIENTED_EDGE('',*,*,#7562,.T.);
#10353=ORIENTED_EDGE('',*,*,#7559,.T.);
#10354=ORIENTED_EDGE('',*,*,#7556,.T.);
#10355=ORIENTED_EDGE('',*,*,#7553,.T.);
#10356=ORIENTED_EDGE('',*,*,#7550,.T.);
#10357=ORIENTED_EDGE('',*,*,#7547,.T.);
#10358=ORIENTED_EDGE('',*,*,#7544,.T.);
#10359=ORIENTED_EDGE('',*,*,#7541,.T.);
#10360=ORIENTED_EDGE('',*,*,#7538,.T.);
#10361=ORIENTED_EDGE('',*,*,#7535,.T.);
#10362=ORIENTED_EDGE('',*,*,#7532,.T.);
#10363=ORIENTED_EDGE('',*,*,#7529,.T.);
#10364=ORIENTED_EDGE('',*,*,#7526,.T.);
#10365=ORIENTED_EDGE('',*,*,#7523,.T.);
#10366=ORIENTED_EDGE('',*,*,#7520,.T.);
#10367=ORIENTED_EDGE('',*,*,#7517,.T.);
#10368=ORIENTED_EDGE('',*,*,#7514,.T.);
#10369=ORIENTED_EDGE('',*,*,#7511,.T.);
#10370=ORIENTED_EDGE('',*,*,#7508,.T.);
#10371=ORIENTED_EDGE('',*,*,#7505,.T.);
#10372=ORIENTED_EDGE('',*,*,#7502,.T.);
#10373=ORIENTED_EDGE('',*,*,#7499,.T.);
#10374=ORIENTED_EDGE('',*,*,#7496,.T.);
#10375=ORIENTED_EDGE('',*,*,#7493,.T.);
#10376=ORIENTED_EDGE('',*,*,#7490,.T.);
#10377=ORIENTED_EDGE('',*,*,#7487,.T.);
#10378=ORIENTED_EDGE('',*,*,#7484,.T.);
#10379=ORIENTED_EDGE('',*,*,#7481,.T.);
#10380=ORIENTED_EDGE('',*,*,#7478,.T.);
#10381=ORIENTED_EDGE('',*,*,#7475,.T.);
#10382=ORIENTED_EDGE('',*,*,#7472,.T.);
#10383=ORIENTED_EDGE('',*,*,#7469,.T.);
#10384=ORIENTED_EDGE('',*,*,#7466,.T.);
#10385=ORIENTED_EDGE('',*,*,#7463,.T.);
#10386=ORIENTED_EDGE('',*,*,#7460,.T.);
#10387=ORIENTED_EDGE('',*,*,#7457,.T.);
#10388=ORIENTED_EDGE('',*,*,#7454,.T.);
#10389=ORIENTED_EDGE('',*,*,#7451,.T.);
#10390=ORIENTED_EDGE('',*,*,#7448,.T.);
#10391=ORIENTED_EDGE('',*,*,#7445,.T.);
#10392=ORIENTED_EDGE('',*,*,#7442,.T.);
#10393=ORIENTED_EDGE('',*,*,#7439,.T.);
#10394=ORIENTED_EDGE('',*,*,#7436,.T.);
#10395=ORIENTED_EDGE('',*,*,#7433,.T.);
#10396=ORIENTED_EDGE('',*,*,#7430,.T.);
#10397=ORIENTED_EDGE('',*,*,#7427,.T.);
#10398=ORIENTED_EDGE('',*,*,#7424,.T.);
#10399=ORIENTED_EDGE('',*,*,#7421,.T.);
#10400=ORIENTED_EDGE('',*,*,#7418,.T.);
#10401=ORIENTED_EDGE('',*,*,#7415,.T.);
#10402=ORIENTED_EDGE('',*,*,#7412,.T.);
#10403=ORIENTED_EDGE('',*,*,#7409,.T.);
#10404=ORIENTED_EDGE('',*,*,#7406,.T.);
#10405=ORIENTED_EDGE('',*,*,#7403,.T.);
#10406=ORIENTED_EDGE('',*,*,#7400,.T.);
#10407=ORIENTED_EDGE('',*,*,#7397,.T.);
#10408=ORIENTED_EDGE('',*,*,#7394,.T.);
#10409=ORIENTED_EDGE('',*,*,#7391,.T.);
#10410=ORIENTED_EDGE('',*,*,#7388,.T.);
#10411=ORIENTED_EDGE('',*,*,#7385,.T.);
#10412=ORIENTED_EDGE('',*,*,#7382,.T.);
#10413=ORIENTED_EDGE('',*,*,#7379,.T.);
#10414=ORIENTED_EDGE('',*,*,#7376,.T.);
#10415=ORIENTED_EDGE('',*,*,#7373,.T.);
#10416=ORIENTED_EDGE('',*,*,#7370,.T.);
#10417=ORIENTED_EDGE('',*,*,#7367,.T.);
#10418=ORIENTED_EDGE('',*,*,#7364,.T.);
#10419=ORIENTED_EDGE('',*,*,#7361,.T.);
#10420=ORIENTED_EDGE('',*,*,#7358,.T.);
#10421=ORIENTED_EDGE('',*,*,#7355,.T.);
#10422=ORIENTED_EDGE('',*,*,#7352,.T.);
#10423=ORIENTED_EDGE('',*,*,#7349,.T.);
#10424=ORIENTED_EDGE('',*,*,#7346,.T.);
#10425=ORIENTED_EDGE('',*,*,#7343,.T.);
#10426=ORIENTED_EDGE('',*,*,#7340,.T.);
#10427=ORIENTED_EDGE('',*,*,#7337,.T.);
#10428=ORIENTED_EDGE('',*,*,#7334,.T.);
#10429=ORIENTED_EDGE('',*,*,#7331,.T.);
#10430=ORIENTED_EDGE('',*,*,#7328,.T.);
#10431=ORIENTED_EDGE('',*,*,#7325,.T.);
#10432=ORIENTED_EDGE('',*,*,#7320,.T.);
#10433=ORIENTED_EDGE('',*,*,#7312,.T.);
#10434=ORIENTED_EDGE('',*,*,#7317,.T.);
#10435=ORIENTED_EDGE('',*,*,#7804,.T.);
#10436=ORIENTED_EDGE('',*,*,#7315,.T.);
#10437=ORIENTED_EDGE('',*,*,#7308,.T.);
#10438=ORIENTED_EDGE('',*,*,#7322,.T.);
#10439=ORIENTED_EDGE('',*,*,#7324,.T.);
#10440=ORIENTED_EDGE('',*,*,#7327,.T.);
#10441=ORIENTED_EDGE('',*,*,#7330,.T.);
#10442=ORIENTED_EDGE('',*,*,#7333,.T.);
#10443=ORIENTED_EDGE('',*,*,#7336,.T.);
#10444=ORIENTED_EDGE('',*,*,#7339,.T.);
#10445=ORIENTED_EDGE('',*,*,#7342,.T.);
#10446=ORIENTED_EDGE('',*,*,#7345,.T.);
#10447=ORIENTED_EDGE('',*,*,#7348,.T.);
#10448=ORIENTED_EDGE('',*,*,#7351,.T.);
#10449=ORIENTED_EDGE('',*,*,#7354,.T.);
#10450=ORIENTED_EDGE('',*,*,#7357,.T.);
#10451=ORIENTED_EDGE('',*,*,#7360,.T.);
#10452=ORIENTED_EDGE('',*,*,#7363,.T.);
#10453=ORIENTED_EDGE('',*,*,#7366,.T.);
#10454=ORIENTED_EDGE('',*,*,#7369,.T.);
#10455=ORIENTED_EDGE('',*,*,#7372,.T.);
#10456=ORIENTED_EDGE('',*,*,#7375,.T.);
#10457=ORIENTED_EDGE('',*,*,#7378,.T.);
#10458=ORIENTED_EDGE('',*,*,#7381,.T.);
#10459=ORIENTED_EDGE('',*,*,#7384,.T.);
#10460=ORIENTED_EDGE('',*,*,#7387,.T.);
#10461=ORIENTED_EDGE('',*,*,#7390,.T.);
#10462=ORIENTED_EDGE('',*,*,#7393,.T.);
#10463=ORIENTED_EDGE('',*,*,#7396,.T.);
#10464=ORIENTED_EDGE('',*,*,#7399,.T.);
#10465=ORIENTED_EDGE('',*,*,#7402,.T.);
#10466=ORIENTED_EDGE('',*,*,#7405,.T.);
#10467=ORIENTED_EDGE('',*,*,#7408,.T.);
#10468=ORIENTED_EDGE('',*,*,#7411,.T.);
#10469=ORIENTED_EDGE('',*,*,#7414,.T.);
#10470=ORIENTED_EDGE('',*,*,#7417,.T.);
#10471=ORIENTED_EDGE('',*,*,#7420,.T.);
#10472=ORIENTED_EDGE('',*,*,#7423,.T.);
#10473=ORIENTED_EDGE('',*,*,#7426,.T.);
#10474=ORIENTED_EDGE('',*,*,#7429,.T.);
#10475=ORIENTED_EDGE('',*,*,#7432,.T.);
#10476=ORIENTED_EDGE('',*,*,#7435,.T.);
#10477=ORIENTED_EDGE('',*,*,#7438,.T.);
#10478=ORIENTED_EDGE('',*,*,#7441,.T.);
#10479=ORIENTED_EDGE('',*,*,#7444,.T.);
#10480=ORIENTED_EDGE('',*,*,#7447,.T.);
#10481=ORIENTED_EDGE('',*,*,#7450,.T.);
#10482=ORIENTED_EDGE('',*,*,#7453,.T.);
#10483=ORIENTED_EDGE('',*,*,#7456,.T.);
#10484=ORIENTED_EDGE('',*,*,#7459,.T.);
#10485=ORIENTED_EDGE('',*,*,#7462,.T.);
#10486=ORIENTED_EDGE('',*,*,#7465,.T.);
#10487=ORIENTED_EDGE('',*,*,#7468,.T.);
#10488=ORIENTED_EDGE('',*,*,#7471,.T.);
#10489=ORIENTED_EDGE('',*,*,#7474,.T.);
#10490=ORIENTED_EDGE('',*,*,#7477,.T.);
#10491=ORIENTED_EDGE('',*,*,#7480,.T.);
#10492=ORIENTED_EDGE('',*,*,#7483,.T.);
#10493=ORIENTED_EDGE('',*,*,#7486,.T.);
#10494=ORIENTED_EDGE('',*,*,#7489,.T.);
#10495=ORIENTED_EDGE('',*,*,#7492,.T.);
#10496=ORIENTED_EDGE('',*,*,#7495,.T.);
#10497=ORIENTED_EDGE('',*,*,#7498,.T.);
#10498=ORIENTED_EDGE('',*,*,#7501,.T.);
#10499=ORIENTED_EDGE('',*,*,#7504,.T.);
#10500=ORIENTED_EDGE('',*,*,#7507,.T.);
#10501=ORIENTED_EDGE('',*,*,#7510,.T.);
#10502=ORIENTED_EDGE('',*,*,#7513,.T.);
#10503=ORIENTED_EDGE('',*,*,#7516,.T.);
#10504=ORIENTED_EDGE('',*,*,#7519,.T.);
#10505=ORIENTED_EDGE('',*,*,#7522,.T.);
#10506=ORIENTED_EDGE('',*,*,#7525,.T.);
#10507=ORIENTED_EDGE('',*,*,#7528,.T.);
#10508=ORIENTED_EDGE('',*,*,#7531,.T.);
#10509=ORIENTED_EDGE('',*,*,#7534,.T.);
#10510=ORIENTED_EDGE('',*,*,#7537,.T.);
#10511=ORIENTED_EDGE('',*,*,#7540,.T.);
#10512=ORIENTED_EDGE('',*,*,#7543,.T.);
#10513=ORIENTED_EDGE('',*,*,#7546,.T.);
#10514=ORIENTED_EDGE('',*,*,#7549,.T.);
#10515=ORIENTED_EDGE('',*,*,#7552,.T.);
#10516=ORIENTED_EDGE('',*,*,#7555,.T.);
#10517=ORIENTED_EDGE('',*,*,#7558,.T.);
#10518=ORIENTED_EDGE('',*,*,#7561,.T.);
#10519=ORIENTED_EDGE('',*,*,#7564,.T.);
#10520=ORIENTED_EDGE('',*,*,#7567,.T.);
#10521=ORIENTED_EDGE('',*,*,#7570,.T.);
#10522=ORIENTED_EDGE('',*,*,#7573,.T.);
#10523=ORIENTED_EDGE('',*,*,#7576,.T.);
#10524=ORIENTED_EDGE('',*,*,#7579,.T.);
#10525=ORIENTED_EDGE('',*,*,#7582,.T.);
#10526=ORIENTED_EDGE('',*,*,#7585,.T.);
#10527=ORIENTED_EDGE('',*,*,#7588,.T.);
#10528=ORIENTED_EDGE('',*,*,#7591,.T.);
#10529=ORIENTED_EDGE('',*,*,#7594,.T.);
#10530=ORIENTED_EDGE('',*,*,#7597,.T.);
#10531=ORIENTED_EDGE('',*,*,#7600,.T.);
#10532=ORIENTED_EDGE('',*,*,#7603,.T.);
#10533=ORIENTED_EDGE('',*,*,#7606,.T.);
#10534=ORIENTED_EDGE('',*,*,#7609,.T.);
#10535=ORIENTED_EDGE('',*,*,#7612,.T.);
#10536=ORIENTED_EDGE('',*,*,#7615,.T.);
#10537=ORIENTED_EDGE('',*,*,#7618,.T.);
#10538=ORIENTED_EDGE('',*,*,#7621,.T.);
#10539=ORIENTED_EDGE('',*,*,#7624,.T.);
#10540=ORIENTED_EDGE('',*,*,#7627,.T.);
#10541=ORIENTED_EDGE('',*,*,#7630,.T.);
#10542=ORIENTED_EDGE('',*,*,#7633,.T.);
#10543=ORIENTED_EDGE('',*,*,#7636,.T.);
#10544=ORIENTED_EDGE('',*,*,#7639,.T.);
#10545=ORIENTED_EDGE('',*,*,#7642,.T.);
#10546=ORIENTED_EDGE('',*,*,#7645,.T.);
#10547=ORIENTED_EDGE('',*,*,#7648,.T.);
#10548=ORIENTED_EDGE('',*,*,#7651,.T.);
#10549=ORIENTED_EDGE('',*,*,#7654,.T.);
#10550=ORIENTED_EDGE('',*,*,#7657,.T.);
#10551=ORIENTED_EDGE('',*,*,#7660,.T.);
#10552=ORIENTED_EDGE('',*,*,#7663,.T.);
#10553=ORIENTED_EDGE('',*,*,#7666,.T.);
#10554=ORIENTED_EDGE('',*,*,#7669,.T.);
#10555=ORIENTED_EDGE('',*,*,#7672,.T.);
#10556=ORIENTED_EDGE('',*,*,#7675,.T.);
#10557=ORIENTED_EDGE('',*,*,#7678,.T.);
#10558=ORIENTED_EDGE('',*,*,#7681,.T.);
#10559=ORIENTED_EDGE('',*,*,#7684,.T.);
#10560=ORIENTED_EDGE('',*,*,#7687,.T.);
#10561=ORIENTED_EDGE('',*,*,#7690,.T.);
#10562=ORIENTED_EDGE('',*,*,#7693,.T.);
#10563=ORIENTED_EDGE('',*,*,#7696,.T.);
#10564=ORIENTED_EDGE('',*,*,#7699,.T.);
#10565=ORIENTED_EDGE('',*,*,#7702,.T.);
#10566=ORIENTED_EDGE('',*,*,#7705,.T.);
#10567=ORIENTED_EDGE('',*,*,#7708,.T.);
#10568=ORIENTED_EDGE('',*,*,#7711,.T.);
#10569=ORIENTED_EDGE('',*,*,#7714,.T.);
#10570=ORIENTED_EDGE('',*,*,#7717,.T.);
#10571=ORIENTED_EDGE('',*,*,#7720,.T.);
#10572=ORIENTED_EDGE('',*,*,#7723,.T.);
#10573=ORIENTED_EDGE('',*,*,#7726,.T.);
#10574=ORIENTED_EDGE('',*,*,#7729,.T.);
#10575=ORIENTED_EDGE('',*,*,#7732,.T.);
#10576=ORIENTED_EDGE('',*,*,#7735,.T.);
#10577=ORIENTED_EDGE('',*,*,#7738,.T.);
#10578=ORIENTED_EDGE('',*,*,#7741,.T.);
#10579=ORIENTED_EDGE('',*,*,#7744,.T.);
#10580=ORIENTED_EDGE('',*,*,#7747,.T.);
#10581=ORIENTED_EDGE('',*,*,#7750,.T.);
#10582=ORIENTED_EDGE('',*,*,#7753,.T.);
#10583=ORIENTED_EDGE('',*,*,#7756,.T.);
#10584=ORIENTED_EDGE('',*,*,#7759,.T.);
#10585=ORIENTED_EDGE('',*,*,#7762,.T.);
#10586=ORIENTED_EDGE('',*,*,#7765,.T.);
#10587=ORIENTED_EDGE('',*,*,#7768,.T.);
#10588=ORIENTED_EDGE('',*,*,#7771,.T.);
#10589=ORIENTED_EDGE('',*,*,#7774,.T.);
#10590=ORIENTED_EDGE('',*,*,#7777,.T.);
#10591=ORIENTED_EDGE('',*,*,#7780,.T.);
#10592=ORIENTED_EDGE('',*,*,#7783,.T.);
#10593=ORIENTED_EDGE('',*,*,#7786,.T.);
#10594=ORIENTED_EDGE('',*,*,#7789,.T.);
#10595=ORIENTED_EDGE('',*,*,#7792,.T.);
#10596=ORIENTED_EDGE('',*,*,#7795,.T.);
#10597=ORIENTED_EDGE('',*,*,#7798,.T.);
#10598=ORIENTED_EDGE('',*,*,#7801,.T.);
#10599=ORIENTED_EDGE('',*,*,#7806,.F.);
#10600=ORIENTED_EDGE('',*,*,#7807,.T.);
#10601=ORIENTED_EDGE('',*,*,#7323,.T.);
#10602=ORIENTED_EDGE('',*,*,#7306,.T.);
#10603=ORIENTED_EDGE('',*,*,#7314,.T.);
#10604=ORIENTED_EDGE('',*,*,#7808,.T.);
#10605=ORIENTED_EDGE('',*,*,#7809,.T.);
#10606=ORIENTED_EDGE('',*,*,#7808,.F.);
#10607=ORIENTED_EDGE('',*,*,#7318,.T.);
#10608=ORIENTED_EDGE('',*,*,#7310,.T.);
#10609=ORIENTED_EDGE('',*,*,#7319,.T.);
#10610=ORIENTED_EDGE('',*,*,#7807,.F.);
#10611=ORIENTED_EDGE('',*,*,#7806,.T.);
#10612=ORIENTED_EDGE('',*,*,#7809,.F.);
#10613=ORIENTED_EDGE('',*,*,#7303,.T.);
#11743=CYLINDRICAL_SURFACE('',#13568,0.425);
#11744=CYLINDRICAL_SURFACE('',#13743,1.);
#12085=ADVANCED_FACE('',(#1576),#11743,.F.);
#12086=ADVANCED_FACE('',(#1577),#1004,.F.);
#12087=ADVANCED_FACE('',(#1578),#1005,.T.);
#12088=ADVANCED_FACE('',(#1579),#1006,.T.);
#12089=ADVANCED_FACE('',(#1580),#1007,.T.);
#12090=ADVANCED_FACE('',(#1581),#1008,.T.);
#12091=ADVANCED_FACE('',(#1582),#1009,.T.);
#12092=ADVANCED_FACE('',(#1583),#1010,.T.);
#12093=ADVANCED_FACE('',(#1584),#1011,.T.);
#12094=ADVANCED_FACE('',(#1585),#1012,.T.);
#12095=ADVANCED_FACE('',(#1586),#1013,.T.);
#12096=ADVANCED_FACE('',(#1587),#1014,.T.);
#12097=ADVANCED_FACE('',(#1588),#1015,.T.);
#12098=ADVANCED_FACE('',(#1589),#1016,.T.);
#12099=ADVANCED_FACE('',(#1590),#1017,.T.);
#12100=ADVANCED_FACE('',(#1591),#1018,.T.);
#12101=ADVANCED_FACE('',(#1592),#1019,.T.);
#12102=ADVANCED_FACE('',(#1593),#1020,.T.);
#12103=ADVANCED_FACE('',(#1594),#1021,.T.);
#12104=ADVANCED_FACE('',(#1595),#1022,.T.);
#12105=ADVANCED_FACE('',(#1596),#1023,.T.);
#12106=ADVANCED_FACE('',(#1597),#1024,.T.);
#12107=ADVANCED_FACE('',(#1598),#1025,.T.);
#12108=ADVANCED_FACE('',(#1599),#1026,.T.);
#12109=ADVANCED_FACE('',(#1600),#1027,.T.);
#12110=ADVANCED_FACE('',(#1601),#1028,.T.);
#12111=ADVANCED_FACE('',(#1602),#1029,.T.);
#12112=ADVANCED_FACE('',(#1603),#1030,.T.);
#12113=ADVANCED_FACE('',(#1604),#1031,.T.);
#12114=ADVANCED_FACE('',(#1605),#1032,.T.);
#12115=ADVANCED_FACE('',(#1606),#1033,.T.);
#12116=ADVANCED_FACE('',(#1607),#1034,.T.);
#12117=ADVANCED_FACE('',(#1608),#1035,.T.);
#12118=ADVANCED_FACE('',(#1609),#1036,.T.);
#12119=ADVANCED_FACE('',(#1610),#1037,.T.);
#12120=ADVANCED_FACE('',(#1611),#1038,.T.);
#12121=ADVANCED_FACE('',(#1612),#1039,.T.);
#12122=ADVANCED_FACE('',(#1613),#1040,.T.);
#12123=ADVANCED_FACE('',(#1614),#1041,.T.);
#12124=ADVANCED_FACE('',(#1615),#1042,.T.);
#12125=ADVANCED_FACE('',(#1616),#1043,.T.);
#12126=ADVANCED_FACE('',(#1617),#1044,.T.);
#12127=ADVANCED_FACE('',(#1618),#1045,.T.);
#12128=ADVANCED_FACE('',(#1619),#1046,.T.);
#12129=ADVANCED_FACE('',(#1620),#1047,.T.);
#12130=ADVANCED_FACE('',(#1621),#1048,.T.);
#12131=ADVANCED_FACE('',(#1622),#1049,.T.);
#12132=ADVANCED_FACE('',(#1623),#1050,.T.);
#12133=ADVANCED_FACE('',(#1624),#1051,.T.);
#12134=ADVANCED_FACE('',(#1625),#1052,.T.);
#12135=ADVANCED_FACE('',(#1626),#1053,.T.);
#12136=ADVANCED_FACE('',(#1627),#1054,.T.);
#12137=ADVANCED_FACE('',(#1628),#1055,.T.);
#12138=ADVANCED_FACE('',(#1629),#1056,.T.);
#12139=ADVANCED_FACE('',(#1630),#1057,.T.);
#12140=ADVANCED_FACE('',(#1631),#1058,.T.);
#12141=ADVANCED_FACE('',(#1632),#1059,.T.);
#12142=ADVANCED_FACE('',(#1633),#1060,.T.);
#12143=ADVANCED_FACE('',(#1634),#1061,.T.);
#12144=ADVANCED_FACE('',(#1635),#1062,.T.);
#12145=ADVANCED_FACE('',(#1636),#1063,.T.);
#12146=ADVANCED_FACE('',(#1637),#1064,.T.);
#12147=ADVANCED_FACE('',(#1638),#1065,.T.);
#12148=ADVANCED_FACE('',(#1639),#1066,.T.);
#12149=ADVANCED_FACE('',(#1640),#1067,.T.);
#12150=ADVANCED_FACE('',(#1641),#1068,.T.);
#12151=ADVANCED_FACE('',(#1642),#1069,.T.);
#12152=ADVANCED_FACE('',(#1643),#1070,.T.);
#12153=ADVANCED_FACE('',(#1644),#1071,.T.);
#12154=ADVANCED_FACE('',(#1645),#1072,.T.);
#12155=ADVANCED_FACE('',(#1646),#1073,.T.);
#12156=ADVANCED_FACE('',(#1647),#1074,.T.);
#12157=ADVANCED_FACE('',(#1648),#1075,.T.);
#12158=ADVANCED_FACE('',(#1649),#1076,.T.);
#12159=ADVANCED_FACE('',(#1650),#1077,.T.);
#12160=ADVANCED_FACE('',(#1651),#1078,.T.);
#12161=ADVANCED_FACE('',(#1652),#1079,.T.);
#12162=ADVANCED_FACE('',(#1653),#1080,.T.);
#12163=ADVANCED_FACE('',(#1654),#1081,.T.);
#12164=ADVANCED_FACE('',(#1655),#1082,.T.);
#12165=ADVANCED_FACE('',(#1656),#1083,.T.);
#12166=ADVANCED_FACE('',(#1657),#1084,.T.);
#12167=ADVANCED_FACE('',(#1658),#1085,.T.);
#12168=ADVANCED_FACE('',(#1659),#1086,.T.);
#12169=ADVANCED_FACE('',(#1660),#1087,.T.);
#12170=ADVANCED_FACE('',(#1661),#1088,.T.);
#12171=ADVANCED_FACE('',(#1662),#1089,.T.);
#12172=ADVANCED_FACE('',(#1663),#1090,.T.);
#12173=ADVANCED_FACE('',(#1664),#1091,.T.);
#12174=ADVANCED_FACE('',(#1665),#1092,.T.);
#12175=ADVANCED_FACE('',(#1666),#1093,.T.);
#12176=ADVANCED_FACE('',(#1667),#1094,.T.);
#12177=ADVANCED_FACE('',(#1668),#1095,.T.);
#12178=ADVANCED_FACE('',(#1669),#1096,.T.);
#12179=ADVANCED_FACE('',(#1670),#1097,.T.);
#12180=ADVANCED_FACE('',(#1671),#1098,.T.);
#12181=ADVANCED_FACE('',(#1672),#1099,.T.);
#12182=ADVANCED_FACE('',(#1673),#1100,.T.);
#12183=ADVANCED_FACE('',(#1674),#1101,.T.);
#12184=ADVANCED_FACE('',(#1675),#1102,.T.);
#12185=ADVANCED_FACE('',(#1676),#1103,.T.);
#12186=ADVANCED_FACE('',(#1677),#1104,.T.);
#12187=ADVANCED_FACE('',(#1678),#1105,.T.);
#12188=ADVANCED_FACE('',(#1679),#1106,.T.);
#12189=ADVANCED_FACE('',(#1680),#1107,.T.);
#12190=ADVANCED_FACE('',(#1681),#1108,.T.);
#12191=ADVANCED_FACE('',(#1682),#1109,.T.);
#12192=ADVANCED_FACE('',(#1683),#1110,.T.);
#12193=ADVANCED_FACE('',(#1684),#1111,.T.);
#12194=ADVANCED_FACE('',(#1685),#1112,.T.);
#12195=ADVANCED_FACE('',(#1686),#1113,.T.);
#12196=ADVANCED_FACE('',(#1687),#1114,.T.);
#12197=ADVANCED_FACE('',(#1688),#1115,.T.);
#12198=ADVANCED_FACE('',(#1689),#1116,.T.);
#12199=ADVANCED_FACE('',(#1690),#1117,.T.);
#12200=ADVANCED_FACE('',(#1691),#1118,.T.);
#12201=ADVANCED_FACE('',(#1692),#1119,.T.);
#12202=ADVANCED_FACE('',(#1693),#1120,.T.);
#12203=ADVANCED_FACE('',(#1694),#1121,.T.);
#12204=ADVANCED_FACE('',(#1695),#1122,.T.);
#12205=ADVANCED_FACE('',(#1696),#1123,.T.);
#12206=ADVANCED_FACE('',(#1697),#1124,.T.);
#12207=ADVANCED_FACE('',(#1698),#1125,.T.);
#12208=ADVANCED_FACE('',(#1699),#1126,.T.);
#12209=ADVANCED_FACE('',(#1700),#1127,.T.);
#12210=ADVANCED_FACE('',(#1701),#1128,.T.);
#12211=ADVANCED_FACE('',(#1702),#1129,.T.);
#12212=ADVANCED_FACE('',(#1703),#1130,.T.);
#12213=ADVANCED_FACE('',(#1704),#1131,.T.);
#12214=ADVANCED_FACE('',(#1705),#1132,.T.);
#12215=ADVANCED_FACE('',(#1706),#1133,.T.);
#12216=ADVANCED_FACE('',(#1707),#1134,.T.);
#12217=ADVANCED_FACE('',(#1708),#1135,.T.);
#12218=ADVANCED_FACE('',(#1709),#1136,.T.);
#12219=ADVANCED_FACE('',(#1710),#1137,.T.);
#12220=ADVANCED_FACE('',(#1711),#1138,.T.);
#12221=ADVANCED_FACE('',(#1712),#1139,.T.);
#12222=ADVANCED_FACE('',(#1713),#1140,.T.);
#12223=ADVANCED_FACE('',(#1714),#1141,.T.);
#12224=ADVANCED_FACE('',(#1715),#1142,.T.);
#12225=ADVANCED_FACE('',(#1716),#1143,.T.);
#12226=ADVANCED_FACE('',(#1717),#1144,.T.);
#12227=ADVANCED_FACE('',(#1718),#1145,.T.);
#12228=ADVANCED_FACE('',(#1719),#1146,.T.);
#12229=ADVANCED_FACE('',(#1720),#1147,.T.);
#12230=ADVANCED_FACE('',(#1721),#1148,.T.);
#12231=ADVANCED_FACE('',(#1722),#1149,.T.);
#12232=ADVANCED_FACE('',(#1723),#1150,.T.);
#12233=ADVANCED_FACE('',(#1724),#1151,.T.);
#12234=ADVANCED_FACE('',(#1725),#1152,.T.);
#12235=ADVANCED_FACE('',(#1726),#1153,.T.);
#12236=ADVANCED_FACE('',(#1727),#1154,.T.);
#12237=ADVANCED_FACE('',(#1728),#1155,.T.);
#12238=ADVANCED_FACE('',(#1729),#1156,.T.);
#12239=ADVANCED_FACE('',(#1730),#1157,.T.);
#12240=ADVANCED_FACE('',(#1731),#1158,.T.);
#12241=ADVANCED_FACE('',(#1732),#1159,.T.);
#12242=ADVANCED_FACE('',(#1733),#1160,.T.);
#12243=ADVANCED_FACE('',(#1734),#1161,.T.);
#12244=ADVANCED_FACE('',(#1735),#1162,.T.);
#12245=ADVANCED_FACE('',(#1736),#1163,.T.);
#12246=ADVANCED_FACE('',(#1737),#1164,.T.);
#12247=ADVANCED_FACE('',(#1738),#1165,.T.);
#12248=ADVANCED_FACE('',(#1739),#1166,.T.);
#12249=ADVANCED_FACE('',(#1740),#1167,.T.);
#12250=ADVANCED_FACE('',(#1741),#1168,.T.);
#12251=ADVANCED_FACE('',(#1742),#1169,.T.);
#12252=ADVANCED_FACE('',(#1743),#1170,.T.);
#12253=ADVANCED_FACE('',(#1744),#1171,.F.);
#12254=ADVANCED_FACE('',(#1745),#11744,.T.);
#12255=ADVANCED_FACE('',(#1746),#1172,.T.);
#12256=ADVANCED_FACE('',(#1747,#812),#1173,.F.);
#12514=CLOSED_SHELL('',(#12085,#12086,#12087,#12088,#12089,#12090,#12091,
#12092,#12093,#12094,#12095,#12096,#12097,#12098,#12099,#12100,#12101,#12102,
#12103,#12104,#12105,#12106,#12107,#12108,#12109,#12110,#12111,#12112,#12113,
#12114,#12115,#12116,#12117,#12118,#12119,#12120,#12121,#12122,#12123,#12124,
#12125,#12126,#12127,#12128,#12129,#12130,#12131,#12132,#12133,#12134,#12135,
#12136,#12137,#12138,#12139,#12140,#12141,#12142,#12143,#12144,#12145,#12146,
#12147,#12148,#12149,#12150,#12151,#12152,#12153,#12154,#12155,#12156,#12157,
#12158,#12159,#12160,#12161,#12162,#12163,#12164,#12165,#12166,#12167,#12168,
#12169,#12170,#12171,#12172,#12173,#12174,#12175,#12176,#12177,#12178,#12179,
#12180,#12181,#12182,#12183,#12184,#12185,#12186,#12187,#12188,#12189,#12190,
#12191,#12192,#12193,#12194,#12195,#12196,#12197,#12198,#12199,#12200,#12201,
#12202,#12203,#12204,#12205,#12206,#12207,#12208,#12209,#12210,#12211,#12212,
#12213,#12214,#12215,#12216,#12217,#12218,#12219,#12220,#12221,#12222,#12223,
#12224,#12225,#12226,#12227,#12228,#12229,#12230,#12231,#12232,#12233,#12234,
#12235,#12236,#12237,#12238,#12239,#12240,#12241,#12242,#12243,#12244,#12245,
#12246,#12247,#12248,#12249,#12250,#12251,#12252,#12253,#12254,#12255,#12256));
#13567=AXIS2_PLACEMENT_3D('',#19315,#15661,#15662);
#13568=AXIS2_PLACEMENT_3D('',#19316,#15663,#15664);
#13569=AXIS2_PLACEMENT_3D('',#19318,#15665,#15666);
#13570=AXIS2_PLACEMENT_3D('',#19321,#15668,#15669);
#13571=AXIS2_PLACEMENT_3D('',#19322,#15670,#15671);
#13572=AXIS2_PLACEMENT_3D('',#19323,#15672,#15673);
#13573=AXIS2_PLACEMENT_3D('',#19332,#15678,#15679);
#13574=AXIS2_PLACEMENT_3D('',#19341,#15684,#15685);
#13575=AXIS2_PLACEMENT_3D('',#19343,#15686,#15687);
#13576=AXIS2_PLACEMENT_3D('',#19349,#15691,#15692);
#13577=AXIS2_PLACEMENT_3D('',#19350,#15693,#15694);
#13578=AXIS2_PLACEMENT_3D('',#19352,#15695,#15696);
#13579=AXIS2_PLACEMENT_3D('',#19358,#15700,#15701);
#13580=AXIS2_PLACEMENT_3D('',#19359,#15702,#15703);
#13581=AXIS2_PLACEMENT_3D('',#19365,#15707,#15708);
#13582=AXIS2_PLACEMENT_3D('',#19371,#15712,#15713);
#13583=AXIS2_PLACEMENT_3D('',#19377,#15717,#15718);
#13584=AXIS2_PLACEMENT_3D('',#19383,#15722,#15723);
#13585=AXIS2_PLACEMENT_3D('',#19389,#15727,#15728);
#13586=AXIS2_PLACEMENT_3D('',#19395,#15732,#15733);
#13587=AXIS2_PLACEMENT_3D('',#19401,#15737,#15738);
#13588=AXIS2_PLACEMENT_3D('',#19407,#15742,#15743);
#13589=AXIS2_PLACEMENT_3D('',#19413,#15747,#15748);
#13590=AXIS2_PLACEMENT_3D('',#19419,#15752,#15753);
#13591=AXIS2_PLACEMENT_3D('',#19425,#15757,#15758);
#13592=AXIS2_PLACEMENT_3D('',#19431,#15762,#15763);
#13593=AXIS2_PLACEMENT_3D('',#19437,#15767,#15768);
#13594=AXIS2_PLACEMENT_3D('',#19443,#15772,#15773);
#13595=AXIS2_PLACEMENT_3D('',#19449,#15777,#15778);
#13596=AXIS2_PLACEMENT_3D('',#19455,#15782,#15783);
#13597=AXIS2_PLACEMENT_3D('',#19461,#15787,#15788);
#13598=AXIS2_PLACEMENT_3D('',#19467,#15792,#15793);
#13599=AXIS2_PLACEMENT_3D('',#19473,#15797,#15798);
#13600=AXIS2_PLACEMENT_3D('',#19479,#15802,#15803);
#13601=AXIS2_PLACEMENT_3D('',#19485,#15807,#15808);
#13602=AXIS2_PLACEMENT_3D('',#19491,#15812,#15813);
#13603=AXIS2_PLACEMENT_3D('',#19497,#15817,#15818);
#13604=AXIS2_PLACEMENT_3D('',#19503,#15822,#15823);
#13605=AXIS2_PLACEMENT_3D('',#19509,#15827,#15828);
#13606=AXIS2_PLACEMENT_3D('',#19515,#15832,#15833);
#13607=AXIS2_PLACEMENT_3D('',#19521,#15837,#15838);
#13608=AXIS2_PLACEMENT_3D('',#19527,#15842,#15843);
#13609=AXIS2_PLACEMENT_3D('',#19533,#15847,#15848);
#13610=AXIS2_PLACEMENT_3D('',#19539,#15852,#15853);
#13611=AXIS2_PLACEMENT_3D('',#19545,#15857,#15858);
#13612=AXIS2_PLACEMENT_3D('',#19551,#15862,#15863);
#13613=AXIS2_PLACEMENT_3D('',#19557,#15867,#15868);
#13614=AXIS2_PLACEMENT_3D('',#19563,#15872,#15873);
#13615=AXIS2_PLACEMENT_3D('',#19569,#15877,#15878);
#13616=AXIS2_PLACEMENT_3D('',#19575,#15882,#15883);
#13617=AXIS2_PLACEMENT_3D('',#19581,#15887,#15888);
#13618=AXIS2_PLACEMENT_3D('',#19587,#15892,#15893);
#13619=AXIS2_PLACEMENT_3D('',#19593,#15897,#15898);
#13620=AXIS2_PLACEMENT_3D('',#19599,#15902,#15903);
#13621=AXIS2_PLACEMENT_3D('',#19605,#15907,#15908);
#13622=AXIS2_PLACEMENT_3D('',#19611,#15912,#15913);
#13623=AXIS2_PLACEMENT_3D('',#19617,#15917,#15918);
#13624=AXIS2_PLACEMENT_3D('',#19623,#15922,#15923);
#13625=AXIS2_PLACEMENT_3D('',#19629,#15927,#15928);
#13626=AXIS2_PLACEMENT_3D('',#19635,#15932,#15933);
#13627=AXIS2_PLACEMENT_3D('',#19641,#15937,#15938);
#13628=AXIS2_PLACEMENT_3D('',#19647,#15942,#15943);
#13629=AXIS2_PLACEMENT_3D('',#19653,#15947,#15948);
#13630=AXIS2_PLACEMENT_3D('',#19659,#15952,#15953);
#13631=AXIS2_PLACEMENT_3D('',#19665,#15957,#15958);
#13632=AXIS2_PLACEMENT_3D('',#19671,#15962,#15963);
#13633=AXIS2_PLACEMENT_3D('',#19677,#15967,#15968);
#13634=AXIS2_PLACEMENT_3D('',#19683,#15972,#15973);
#13635=AXIS2_PLACEMENT_3D('',#19689,#15977,#15978);
#13636=AXIS2_PLACEMENT_3D('',#19695,#15982,#15983);
#13637=AXIS2_PLACEMENT_3D('',#19701,#15987,#15988);
#13638=AXIS2_PLACEMENT_3D('',#19707,#15992,#15993);
#13639=AXIS2_PLACEMENT_3D('',#19713,#15997,#15998);
#13640=AXIS2_PLACEMENT_3D('',#19719,#16002,#16003);
#13641=AXIS2_PLACEMENT_3D('',#19725,#16007,#16008);
#13642=AXIS2_PLACEMENT_3D('',#19731,#16012,#16013);
#13643=AXIS2_PLACEMENT_3D('',#19737,#16017,#16018);
#13644=AXIS2_PLACEMENT_3D('',#19743,#16022,#16023);
#13645=AXIS2_PLACEMENT_3D('',#19749,#16027,#16028);
#13646=AXIS2_PLACEMENT_3D('',#19755,#16032,#16033);
#13647=AXIS2_PLACEMENT_3D('',#19761,#16037,#16038);
#13648=AXIS2_PLACEMENT_3D('',#19767,#16042,#16043);
#13649=AXIS2_PLACEMENT_3D('',#19773,#16047,#16048);
#13650=AXIS2_PLACEMENT_3D('',#19779,#16052,#16053);
#13651=AXIS2_PLACEMENT_3D('',#19785,#16057,#16058);
#13652=AXIS2_PLACEMENT_3D('',#19791,#16062,#16063);
#13653=AXIS2_PLACEMENT_3D('',#19797,#16067,#16068);
#13654=AXIS2_PLACEMENT_3D('',#19803,#16072,#16073);
#13655=AXIS2_PLACEMENT_3D('',#19809,#16077,#16078);
#13656=AXIS2_PLACEMENT_3D('',#19815,#16082,#16083);
#13657=AXIS2_PLACEMENT_3D('',#19821,#16087,#16088);
#13658=AXIS2_PLACEMENT_3D('',#19827,#16092,#16093);
#13659=AXIS2_PLACEMENT_3D('',#19833,#16097,#16098);
#13660=AXIS2_PLACEMENT_3D('',#19839,#16102,#16103);
#13661=AXIS2_PLACEMENT_3D('',#19845,#16107,#16108);
#13662=AXIS2_PLACEMENT_3D('',#19851,#16112,#16113);
#13663=AXIS2_PLACEMENT_3D('',#19857,#16117,#16118);
#13664=AXIS2_PLACEMENT_3D('',#19863,#16122,#16123);
#13665=AXIS2_PLACEMENT_3D('',#19869,#16127,#16128);
#13666=AXIS2_PLACEMENT_3D('',#19875,#16132,#16133);
#13667=AXIS2_PLACEMENT_3D('',#19881,#16137,#16138);
#13668=AXIS2_PLACEMENT_3D('',#19887,#16142,#16143);
#13669=AXIS2_PLACEMENT_3D('',#19893,#16147,#16148);
#13670=AXIS2_PLACEMENT_3D('',#19899,#16152,#16153);
#13671=AXIS2_PLACEMENT_3D('',#19905,#16157,#16158);
#13672=AXIS2_PLACEMENT_3D('',#19911,#16162,#16163);
#13673=AXIS2_PLACEMENT_3D('',#19917,#16167,#16168);
#13674=AXIS2_PLACEMENT_3D('',#19923,#16172,#16173);
#13675=AXIS2_PLACEMENT_3D('',#19929,#16177,#16178);
#13676=AXIS2_PLACEMENT_3D('',#19935,#16182,#16183);
#13677=AXIS2_PLACEMENT_3D('',#19941,#16187,#16188);
#13678=AXIS2_PLACEMENT_3D('',#19947,#16192,#16193);
#13679=AXIS2_PLACEMENT_3D('',#19953,#16197,#16198);
#13680=AXIS2_PLACEMENT_3D('',#19959,#16202,#16203);
#13681=AXIS2_PLACEMENT_3D('',#19965,#16207,#16208);
#13682=AXIS2_PLACEMENT_3D('',#19971,#16212,#16213);
#13683=AXIS2_PLACEMENT_3D('',#19977,#16217,#16218);
#13684=AXIS2_PLACEMENT_3D('',#19983,#16222,#16223);
#13685=AXIS2_PLACEMENT_3D('',#19989,#16227,#16228);
#13686=AXIS2_PLACEMENT_3D('',#19995,#16232,#16233);
#13687=AXIS2_PLACEMENT_3D('',#20001,#16237,#16238);
#13688=AXIS2_PLACEMENT_3D('',#20007,#16242,#16243);
#13689=AXIS2_PLACEMENT_3D('',#20013,#16247,#16248);
#13690=AXIS2_PLACEMENT_3D('',#20019,#16252,#16253);
#13691=AXIS2_PLACEMENT_3D('',#20025,#16257,#16258);
#13692=AXIS2_PLACEMENT_3D('',#20031,#16262,#16263);
#13693=AXIS2_PLACEMENT_3D('',#20037,#16267,#16268);
#13694=AXIS2_PLACEMENT_3D('',#20043,#16272,#16273);
#13695=AXIS2_PLACEMENT_3D('',#20049,#16277,#16278);
#13696=AXIS2_PLACEMENT_3D('',#20055,#16282,#16283);
#13697=AXIS2_PLACEMENT_3D('',#20061,#16287,#16288);
#13698=AXIS2_PLACEMENT_3D('',#20067,#16292,#16293);
#13699=AXIS2_PLACEMENT_3D('',#20073,#16297,#16298);
#13700=AXIS2_PLACEMENT_3D('',#20079,#16302,#16303);
#13701=AXIS2_PLACEMENT_3D('',#20085,#16307,#16308);
#13702=AXIS2_PLACEMENT_3D('',#20091,#16312,#16313);
#13703=AXIS2_PLACEMENT_3D('',#20097,#16317,#16318);
#13704=AXIS2_PLACEMENT_3D('',#20103,#16322,#16323);
#13705=AXIS2_PLACEMENT_3D('',#20109,#16327,#16328);
#13706=AXIS2_PLACEMENT_3D('',#20115,#16332,#16333);
#13707=AXIS2_PLACEMENT_3D('',#20121,#16337,#16338);
#13708=AXIS2_PLACEMENT_3D('',#20127,#16342,#16343);
#13709=AXIS2_PLACEMENT_3D('',#20133,#16347,#16348);
#13710=AXIS2_PLACEMENT_3D('',#20139,#16352,#16353);
#13711=AXIS2_PLACEMENT_3D('',#20145,#16357,#16358);
#13712=AXIS2_PLACEMENT_3D('',#20151,#16362,#16363);
#13713=AXIS2_PLACEMENT_3D('',#20157,#16367,#16368);
#13714=AXIS2_PLACEMENT_3D('',#20163,#16372,#16373);
#13715=AXIS2_PLACEMENT_3D('',#20169,#16377,#16378);
#13716=AXIS2_PLACEMENT_3D('',#20175,#16382,#16383);
#13717=AXIS2_PLACEMENT_3D('',#20181,#16387,#16388);
#13718=AXIS2_PLACEMENT_3D('',#20187,#16392,#16393);
#13719=AXIS2_PLACEMENT_3D('',#20193,#16397,#16398);
#13720=AXIS2_PLACEMENT_3D('',#20199,#16402,#16403);
#13721=AXIS2_PLACEMENT_3D('',#20205,#16407,#16408);
#13722=AXIS2_PLACEMENT_3D('',#20211,#16412,#16413);
#13723=AXIS2_PLACEMENT_3D('',#20217,#16417,#16418);
#13724=AXIS2_PLACEMENT_3D('',#20223,#16422,#16423);
#13725=AXIS2_PLACEMENT_3D('',#20229,#16427,#16428);
#13726=AXIS2_PLACEMENT_3D('',#20235,#16432,#16433);
#13727=AXIS2_PLACEMENT_3D('',#20241,#16437,#16438);
#13728=AXIS2_PLACEMENT_3D('',#20247,#16442,#16443);
#13729=AXIS2_PLACEMENT_3D('',#20253,#16447,#16448);
#13730=AXIS2_PLACEMENT_3D('',#20259,#16452,#16453);
#13731=AXIS2_PLACEMENT_3D('',#20265,#16457,#16458);
#13732=AXIS2_PLACEMENT_3D('',#20271,#16462,#16463);
#13733=AXIS2_PLACEMENT_3D('',#20277,#16467,#16468);
#13734=AXIS2_PLACEMENT_3D('',#20283,#16472,#16473);
#13735=AXIS2_PLACEMENT_3D('',#20289,#16477,#16478);
#13736=AXIS2_PLACEMENT_3D('',#20295,#16482,#16483);
#13737=AXIS2_PLACEMENT_3D('',#20301,#16487,#16488);
#13738=AXIS2_PLACEMENT_3D('',#20307,#16492,#16493);
#13739=AXIS2_PLACEMENT_3D('',#20313,#16497,#16498);
#13740=AXIS2_PLACEMENT_3D('',#20319,#16502,#16503);
#13741=AXIS2_PLACEMENT_3D('',#20322,#16506,#16507);
#13742=AXIS2_PLACEMENT_3D('',#20323,#16508,#16509);
#13743=AXIS2_PLACEMENT_3D('',#20324,#16510,#16511);
#13744=AXIS2_PLACEMENT_3D('',#20326,#16512,#16513);
#13745=AXIS2_PLACEMENT_3D('',#20330,#16516,#16517);
#13746=AXIS2_PLACEMENT_3D('',#20331,#16518,#16519);
#13747=AXIS2_PLACEMENT_3D('',#20332,#16520,#16521);
#15661=DIRECTION('axis',(0.,0.,1.));
#15662=DIRECTION('refdir',(1.,0.,0.));
#15663=DIRECTION('center_axis',(0.,0.,1.));
#15664=DIRECTION('ref_axis',(1.,0.,0.));
#15665=DIRECTION('center_axis',(0.,0.,1.));
#15666=DIRECTION('ref_axis',(1.,0.,0.));
#15667=DIRECTION('',(0.,0.,1.));
#15668=DIRECTION('center_axis',(0.,0.,1.));
#15669=DIRECTION('ref_axis',(1.,0.,0.));
#15670=DIRECTION('center_axis',(0.,0.,1.));
#15671=DIRECTION('ref_axis',(1.,0.,0.));
#15672=DIRECTION('center_axis',(1.,0.,0.));
#15673=DIRECTION('ref_axis',(0.,0.,-1.));
#15674=DIRECTION('',(0.,0.,-1.));
#15675=DIRECTION('',(0.,1.,0.));
#15676=DIRECTION('',(0.,0.,1.));
#15677=DIRECTION('',(0.,1.,0.));
#15678=DIRECTION('center_axis',(1.,0.,0.));
#15679=DIRECTION('ref_axis',(0.,0.,-1.));
#15680=DIRECTION('',(0.,0.,1.));
#15681=DIRECTION('',(0.,1.,0.));
#15682=DIRECTION('',(0.,0.,-1.));
#15683=DIRECTION('',(0.,1.,0.));
#15684=DIRECTION('center_axis',(0.,0.,-1.));
#15685=DIRECTION('ref_axis',(-1.,0.,0.));
#15686=DIRECTION('center_axis',(0.,0.,-1.));
#15687=DIRECTION('ref_axis',(1.,0.,0.));
#15688=DIRECTION('',(1.,0.,0.));
#15689=DIRECTION('',(0.,1.,0.));
#15690=DIRECTION('',(-1.,0.,0.));
#15691=DIRECTION('center_axis',(0.,0.,-1.));
#15692=DIRECTION('ref_axis',(1.,0.,0.));
#15693=DIRECTION('center_axis',(0.,0.,1.));
#15694=DIRECTION('ref_axis',(1.,0.,0.));
#15695=DIRECTION('center_axis',(0.,0.,1.));
#15696=DIRECTION('ref_axis',(1.,0.,0.));
#15697=DIRECTION('',(1.,0.,0.));
#15698=DIRECTION('',(0.,1.,0.));
#15699=DIRECTION('',(-1.,0.,0.));
#15700=DIRECTION('center_axis',(0.,0.,1.));
#15701=DIRECTION('ref_axis',(1.,0.,0.));
#15702=DIRECTION('center_axis',(-1.,0.,0.));
#15703=DIRECTION('ref_axis',(0.,0.,1.));
#15704=DIRECTION('',(0.,0.,-1.));
#15705=DIRECTION('',(0.,0.,1.));
#15706=DIRECTION('',(0.,1.,0.));
#15707=DIRECTION('center_axis',(-0.342020143325675,0.,0.939692620785906));
#15708=DIRECTION('ref_axis',(0.939692620785906,0.,0.342020143325675));
#15709=DIRECTION('',(-0.939692620785906,0.,-0.342020143325675));
#15710=DIRECTION('',(0.939692620785906,0.,0.342020143325675));
#15711=DIRECTION('',(0.,1.,0.));
#15712=DIRECTION('center_axis',(-1.,0.,0.));
#15713=DIRECTION('ref_axis',(0.,0.,1.));
#15714=DIRECTION('',(0.,0.,-1.));
#15715=DIRECTION('',(0.,0.,1.));
#15716=DIRECTION('',(0.,1.,0.));
#15717=DIRECTION('center_axis',(-0.342020143325675,0.,-0.939692620785906));
#15718=DIRECTION('ref_axis',(-0.939692620785906,0.,0.342020143325675));
#15719=DIRECTION('',(0.939692620785906,0.,-0.342020143325675));
#15720=DIRECTION('',(-0.939692620785906,0.,0.342020143325675));
#15721=DIRECTION('',(0.,1.,0.));
#15722=DIRECTION('center_axis',(-1.,0.,0.));
#15723=DIRECTION('ref_axis',(0.,0.,1.));
#15724=DIRECTION('',(0.,0.,-1.));
#15725=DIRECTION('',(0.,0.,1.));
#15726=DIRECTION('',(0.,1.,0.));
#15727=DIRECTION('center_axis',(-0.342020143325675,0.,0.939692620785906));
#15728=DIRECTION('ref_axis',(0.939692620785906,0.,0.342020143325675));
#15729=DIRECTION('',(-0.939692620785906,0.,-0.342020143325675));
#15730=DIRECTION('',(0.939692620785906,0.,0.342020143325675));
#15731=DIRECTION('',(0.,1.,0.));
#15732=DIRECTION('center_axis',(-1.,0.,0.));
#15733=DIRECTION('ref_axis',(0.,0.,1.));
#15734=DIRECTION('',(0.,0.,-1.));
#15735=DIRECTION('',(0.,0.,1.));
#15736=DIRECTION('',(0.,1.,0.));
#15737=DIRECTION('center_axis',(-0.342020143325675,0.,-0.939692620785906));
#15738=DIRECTION('ref_axis',(-0.939692620785906,0.,0.342020143325675));
#15739=DIRECTION('',(0.939692620785906,0.,-0.342020143325675));
#15740=DIRECTION('',(-0.939692620785906,0.,0.342020143325675));
#15741=DIRECTION('',(0.,1.,0.));
#15742=DIRECTION('center_axis',(-1.,0.,0.));
#15743=DIRECTION('ref_axis',(0.,0.,1.));
#15744=DIRECTION('',(0.,0.,-1.));
#15745=DIRECTION('',(0.,0.,1.));
#15746=DIRECTION('',(0.,1.,0.));
#15747=DIRECTION('center_axis',(-0.342020143325675,0.,0.939692620785906));
#15748=DIRECTION('ref_axis',(0.939692620785906,0.,0.342020143325675));
#15749=DIRECTION('',(-0.939692620785906,0.,-0.342020143325675));
#15750=DIRECTION('',(0.939692620785906,0.,0.342020143325675));
#15751=DIRECTION('',(0.,1.,0.));
#15752=DIRECTION('center_axis',(-1.,0.,0.));
#15753=DIRECTION('ref_axis',(0.,0.,1.));
#15754=DIRECTION('',(0.,0.,-1.));
#15755=DIRECTION('',(0.,0.,1.));
#15756=DIRECTION('',(0.,1.,0.));
#15757=DIRECTION('center_axis',(-0.342020143325675,0.,-0.939692620785906));
#15758=DIRECTION('ref_axis',(-0.939692620785906,0.,0.342020143325675));
#15759=DIRECTION('',(0.939692620785906,0.,-0.342020143325675));
#15760=DIRECTION('',(-0.939692620785906,0.,0.342020143325675));
#15761=DIRECTION('',(0.,1.,0.));
#15762=DIRECTION('center_axis',(-1.,0.,0.));
#15763=DIRECTION('ref_axis',(0.,0.,1.));
#15764=DIRECTION('',(0.,0.,-1.));
#15765=DIRECTION('',(0.,0.,1.));
#15766=DIRECTION('',(0.,1.,0.));
#15767=DIRECTION('center_axis',(-0.342020143325675,0.,0.939692620785906));
#15768=DIRECTION('ref_axis',(0.939692620785906,0.,0.342020143325675));
#15769=DIRECTION('',(-0.939692620785906,0.,-0.342020143325675));
#15770=DIRECTION('',(0.939692620785906,0.,0.342020143325675));
#15771=DIRECTION('',(0.,1.,0.));
#15772=DIRECTION('center_axis',(-1.,0.,0.));
#15773=DIRECTION('ref_axis',(0.,0.,1.));
#15774=DIRECTION('',(0.,0.,-1.));
#15775=DIRECTION('',(0.,0.,1.));
#15776=DIRECTION('',(0.,1.,0.));
#15777=DIRECTION('center_axis',(-0.342020143325675,0.,-0.939692620785906));
#15778=DIRECTION('ref_axis',(-0.939692620785906,0.,0.342020143325675));
#15779=DIRECTION('',(0.939692620785906,0.,-0.342020143325675));
#15780=DIRECTION('',(-0.939692620785906,0.,0.342020143325675));
#15781=DIRECTION('',(0.,1.,0.));
#15782=DIRECTION('center_axis',(-1.,0.,0.));
#15783=DIRECTION('ref_axis',(0.,0.,1.));
#15784=DIRECTION('',(0.,0.,-1.));
#15785=DIRECTION('',(0.,0.,1.));
#15786=DIRECTION('',(0.,1.,0.));
#15787=DIRECTION('center_axis',(-0.342020143325662,0.,0.939692620785911));
#15788=DIRECTION('ref_axis',(0.939692620785911,0.,0.342020143325662));
#15789=DIRECTION('',(-0.939692620785911,0.,-0.342020143325662));
#15790=DIRECTION('',(0.939692620785911,0.,0.342020143325662));
#15791=DIRECTION('',(0.,1.,0.));
#15792=DIRECTION('center_axis',(-1.,0.,0.));
#15793=DIRECTION('ref_axis',(0.,0.,1.));
#15794=DIRECTION('',(0.,0.,-1.));
#15795=DIRECTION('',(0.,0.,1.));
#15796=DIRECTION('',(0.,1.,0.));
#15797=DIRECTION('center_axis',(-0.342020143325662,0.,-0.939692620785911));
#15798=DIRECTION('ref_axis',(-0.939692620785911,0.,0.342020143325662));
#15799=DIRECTION('',(0.939692620785911,0.,-0.342020143325662));
#15800=DIRECTION('',(-0.939692620785911,0.,0.342020143325662));
#15801=DIRECTION('',(0.,1.,0.));
#15802=DIRECTION('center_axis',(-1.,0.,0.));
#15803=DIRECTION('ref_axis',(0.,0.,1.));
#15804=DIRECTION('',(0.,0.,-1.));
#15805=DIRECTION('',(0.,0.,1.));
#15806=DIRECTION('',(0.,1.,0.));
#15807=DIRECTION('center_axis',(-0.342020143325662,0.,0.939692620785911));
#15808=DIRECTION('ref_axis',(0.939692620785911,0.,0.342020143325662));
#15809=DIRECTION('',(-0.939692620785911,0.,-0.342020143325662));
#15810=DIRECTION('',(0.939692620785911,0.,0.342020143325662));
#15811=DIRECTION('',(0.,1.,0.));
#15812=DIRECTION('center_axis',(-1.,0.,0.));
#15813=DIRECTION('ref_axis',(0.,0.,1.));
#15814=DIRECTION('',(0.,0.,-1.));
#15815=DIRECTION('',(0.,0.,1.));
#15816=DIRECTION('',(0.,1.,0.));
#15817=DIRECTION('center_axis',(-0.342020143325662,0.,-0.939692620785911));
#15818=DIRECTION('ref_axis',(-0.939692620785911,0.,0.342020143325662));
#15819=DIRECTION('',(0.939692620785911,0.,-0.342020143325662));
#15820=DIRECTION('',(-0.939692620785911,0.,0.342020143325662));
#15821=DIRECTION('',(0.,1.,0.));
#15822=DIRECTION('center_axis',(-1.,0.,0.));
#15823=DIRECTION('ref_axis',(0.,0.,1.));
#15824=DIRECTION('',(0.,0.,-1.));
#15825=DIRECTION('',(0.,0.,1.));
#15826=DIRECTION('',(0.,1.,0.));
#15827=DIRECTION('center_axis',(-0.342020143325662,0.,0.939692620785911));
#15828=DIRECTION('ref_axis',(0.939692620785911,0.,0.342020143325662));
#15829=DIRECTION('',(-0.939692620785911,0.,-0.342020143325662));
#15830=DIRECTION('',(0.939692620785911,0.,0.342020143325662));
#15831=DIRECTION('',(0.,1.,0.));
#15832=DIRECTION('center_axis',(-1.,0.,0.));
#15833=DIRECTION('ref_axis',(0.,0.,1.));
#15834=DIRECTION('',(0.,0.,-1.));
#15835=DIRECTION('',(0.,0.,1.));
#15836=DIRECTION('',(0.,1.,0.));
#15837=DIRECTION('center_axis',(-0.342020143325662,0.,-0.939692620785911));
#15838=DIRECTION('ref_axis',(-0.939692620785911,0.,0.342020143325662));
#15839=DIRECTION('',(0.939692620785911,0.,-0.342020143325662));
#15840=DIRECTION('',(-0.939692620785911,0.,0.342020143325662));
#15841=DIRECTION('',(0.,1.,0.));
#15842=DIRECTION('center_axis',(-1.,0.,0.));
#15843=DIRECTION('ref_axis',(0.,0.,1.));
#15844=DIRECTION('',(0.,0.,-1.));
#15845=DIRECTION('',(0.,0.,1.));
#15846=DIRECTION('',(0.,1.,0.));
#15847=DIRECTION('center_axis',(-0.342020143325668,0.,0.939692620785909));
#15848=DIRECTION('ref_axis',(0.939692620785909,0.,0.342020143325668));
#15849=DIRECTION('',(-0.939692620785909,0.,-0.342020143325668));
#15850=DIRECTION('',(0.939692620785909,0.,0.342020143325668));
#15851=DIRECTION('',(0.,1.,0.));
#15852=DIRECTION('center_axis',(-1.,0.,0.));
#15853=DIRECTION('ref_axis',(0.,0.,1.));
#15854=DIRECTION('',(0.,0.,-1.));
#15855=DIRECTION('',(0.,0.,1.));
#15856=DIRECTION('',(0.,1.,0.));
#15857=DIRECTION('center_axis',(-0.342020143325668,0.,-0.939692620785909));
#15858=DIRECTION('ref_axis',(-0.939692620785909,0.,0.342020143325668));
#15859=DIRECTION('',(0.939692620785909,0.,-0.342020143325668));
#15860=DIRECTION('',(-0.939692620785909,0.,0.342020143325668));
#15861=DIRECTION('',(0.,1.,0.));
#15862=DIRECTION('center_axis',(-1.,0.,0.));
#15863=DIRECTION('ref_axis',(0.,0.,1.));
#15864=DIRECTION('',(0.,0.,-1.));
#15865=DIRECTION('',(0.,0.,1.));
#15866=DIRECTION('',(0.,1.,0.));
#15867=DIRECTION('center_axis',(-0.342020143325668,0.,0.939692620785909));
#15868=DIRECTION('ref_axis',(0.939692620785909,0.,0.342020143325668));
#15869=DIRECTION('',(-0.939692620785909,0.,-0.342020143325668));
#15870=DIRECTION('',(0.939692620785909,0.,0.342020143325668));
#15871=DIRECTION('',(0.,1.,0.));
#15872=DIRECTION('center_axis',(-1.,0.,0.));
#15873=DIRECTION('ref_axis',(0.,0.,1.));
#15874=DIRECTION('',(0.,0.,-1.));
#15875=DIRECTION('',(0.,0.,1.));
#15876=DIRECTION('',(0.,1.,0.));
#15877=DIRECTION('center_axis',(-0.342020143325668,0.,-0.939692620785909));
#15878=DIRECTION('ref_axis',(-0.939692620785909,0.,0.342020143325668));
#15879=DIRECTION('',(0.939692620785909,0.,-0.342020143325668));
#15880=DIRECTION('',(-0.939692620785909,0.,0.342020143325668));
#15881=DIRECTION('',(0.,1.,0.));
#15882=DIRECTION('center_axis',(-1.,0.,0.));
#15883=DIRECTION('ref_axis',(0.,0.,1.));
#15884=DIRECTION('',(0.,0.,-1.));
#15885=DIRECTION('',(0.,0.,1.));
#15886=DIRECTION('',(0.,1.,0.));
#15887=DIRECTION('center_axis',(-0.342020143325668,0.,0.939692620785909));
#15888=DIRECTION('ref_axis',(0.939692620785909,0.,0.342020143325668));
#15889=DIRECTION('',(-0.939692620785909,0.,-0.342020143325668));
#15890=DIRECTION('',(0.939692620785909,0.,0.342020143325668));
#15891=DIRECTION('',(0.,1.,0.));
#15892=DIRECTION('center_axis',(-1.,0.,0.));
#15893=DIRECTION('ref_axis',(0.,0.,1.));
#15894=DIRECTION('',(0.,0.,-1.));
#15895=DIRECTION('',(0.,0.,1.));
#15896=DIRECTION('',(0.,1.,0.));
#15897=DIRECTION('center_axis',(-0.342020143325668,0.,-0.939692620785909));
#15898=DIRECTION('ref_axis',(-0.939692620785909,0.,0.342020143325668));
#15899=DIRECTION('',(0.939692620785909,0.,-0.342020143325668));
#15900=DIRECTION('',(-0.939692620785909,0.,0.342020143325668));
#15901=DIRECTION('',(0.,1.,0.));
#15902=DIRECTION('center_axis',(-1.,0.,0.));
#15903=DIRECTION('ref_axis',(0.,0.,1.));
#15904=DIRECTION('',(0.,0.,-1.));
#15905=DIRECTION('',(0.,0.,1.));
#15906=DIRECTION('',(0.,1.,0.));
#15907=DIRECTION('center_axis',(-0.342020143325668,0.,0.939692620785909));
#15908=DIRECTION('ref_axis',(0.939692620785909,0.,0.342020143325668));
#15909=DIRECTION('',(-0.939692620785909,0.,-0.342020143325668));
#15910=DIRECTION('',(0.939692620785909,0.,0.342020143325668));
#15911=DIRECTION('',(0.,1.,0.));
#15912=DIRECTION('center_axis',(-1.,0.,0.));
#15913=DIRECTION('ref_axis',(0.,0.,1.));
#15914=DIRECTION('',(0.,0.,-1.));
#15915=DIRECTION('',(0.,0.,1.));
#15916=DIRECTION('',(0.,1.,0.));
#15917=DIRECTION('center_axis',(-0.342020143325668,0.,-0.939692620785909));
#15918=DIRECTION('ref_axis',(-0.939692620785909,0.,0.342020143325668));
#15919=DIRECTION('',(0.939692620785909,0.,-0.342020143325668));
#15920=DIRECTION('',(-0.939692620785909,0.,0.342020143325668));
#15921=DIRECTION('',(0.,1.,0.));
#15922=DIRECTION('center_axis',(-1.,0.,0.));
#15923=DIRECTION('ref_axis',(0.,0.,1.));
#15924=DIRECTION('',(0.,0.,-1.));
#15925=DIRECTION('',(0.,0.,1.));
#15926=DIRECTION('',(0.,1.,0.));
#15927=DIRECTION('center_axis',(-0.342020143325668,0.,0.939692620785909));
#15928=DIRECTION('ref_axis',(0.939692620785909,0.,0.342020143325668));
#15929=DIRECTION('',(-0.939692620785909,0.,-0.342020143325668));
#15930=DIRECTION('',(0.939692620785909,0.,0.342020143325668));
#15931=DIRECTION('',(0.,1.,0.));
#15932=DIRECTION('center_axis',(-1.,0.,0.));
#15933=DIRECTION('ref_axis',(0.,0.,1.));
#15934=DIRECTION('',(0.,0.,-1.));
#15935=DIRECTION('',(0.,0.,1.));
#15936=DIRECTION('',(0.,1.,0.));
#15937=DIRECTION('center_axis',(-0.342020143325668,0.,-0.939692620785909));
#15938=DIRECTION('ref_axis',(-0.939692620785909,0.,0.342020143325668));
#15939=DIRECTION('',(0.939692620785909,0.,-0.342020143325668));
#15940=DIRECTION('',(-0.939692620785909,0.,0.342020143325668));
#15941=DIRECTION('',(0.,1.,0.));
#15942=DIRECTION('center_axis',(-1.,0.,0.));
#15943=DIRECTION('ref_axis',(0.,0.,1.));
#15944=DIRECTION('',(0.,0.,-1.));
#15945=DIRECTION('',(0.,0.,1.));
#15946=DIRECTION('',(0.,1.,0.));
#15947=DIRECTION('center_axis',(-0.342020143325668,0.,0.939692620785909));
#15948=DIRECTION('ref_axis',(0.939692620785909,0.,0.342020143325668));
#15949=DIRECTION('',(-0.939692620785909,0.,-0.342020143325668));
#15950=DIRECTION('',(0.939692620785909,0.,0.342020143325668));
#15951=DIRECTION('',(0.,1.,0.));
#15952=DIRECTION('center_axis',(-1.,0.,0.));
#15953=DIRECTION('ref_axis',(0.,0.,1.));
#15954=DIRECTION('',(0.,0.,-1.));
#15955=DIRECTION('',(0.,0.,1.));
#15956=DIRECTION('',(0.,1.,0.));
#15957=DIRECTION('center_axis',(-0.342020143325668,0.,-0.939692620785909));
#15958=DIRECTION('ref_axis',(-0.939692620785909,0.,0.342020143325668));
#15959=DIRECTION('',(0.939692620785909,0.,-0.342020143325668));
#15960=DIRECTION('',(-0.939692620785909,0.,0.342020143325668));
#15961=DIRECTION('',(0.,1.,0.));
#15962=DIRECTION('center_axis',(-1.,0.,0.));
#15963=DIRECTION('ref_axis',(0.,0.,1.));
#15964=DIRECTION('',(0.,0.,-1.));
#15965=DIRECTION('',(0.,0.,1.));
#15966=DIRECTION('',(0.,1.,0.));
#15967=DIRECTION('center_axis',(-0.342020143325668,0.,0.939692620785909));
#15968=DIRECTION('ref_axis',(0.939692620785909,0.,0.342020143325668));
#15969=DIRECTION('',(-0.939692620785909,0.,-0.342020143325668));
#15970=DIRECTION('',(0.939692620785909,0.,0.342020143325668));
#15971=DIRECTION('',(0.,1.,0.));
#15972=DIRECTION('center_axis',(-1.,0.,0.));
#15973=DIRECTION('ref_axis',(0.,0.,1.));
#15974=DIRECTION('',(0.,0.,-1.));
#15975=DIRECTION('',(0.,0.,1.));
#15976=DIRECTION('',(0.,1.,0.));
#15977=DIRECTION('center_axis',(-0.342020143325668,0.,-0.939692620785909));
#15978=DIRECTION('ref_axis',(-0.939692620785909,0.,0.342020143325668));
#15979=DIRECTION('',(0.939692620785909,0.,-0.342020143325668));
#15980=DIRECTION('',(-0.939692620785909,0.,0.342020143325668));
#15981=DIRECTION('',(0.,1.,0.));
#15982=DIRECTION('center_axis',(-1.,0.,0.));
#15983=DIRECTION('ref_axis',(0.,0.,1.));
#15984=DIRECTION('',(0.,0.,-1.));
#15985=DIRECTION('',(0.,0.,1.));
#15986=DIRECTION('',(0.,1.,0.));
#15987=DIRECTION('center_axis',(-0.342020143325662,0.,0.939692620785911));
#15988=DIRECTION('ref_axis',(0.939692620785911,0.,0.342020143325662));
#15989=DIRECTION('',(-0.939692620785911,0.,-0.342020143325662));
#15990=DIRECTION('',(0.939692620785911,0.,0.342020143325662));
#15991=DIRECTION('',(0.,1.,0.));
#15992=DIRECTION('center_axis',(-1.,0.,0.));
#15993=DIRECTION('ref_axis',(0.,0.,1.));
#15994=DIRECTION('',(0.,0.,-1.));
#15995=DIRECTION('',(0.,0.,1.));
#15996=DIRECTION('',(0.,1.,0.));
#15997=DIRECTION('center_axis',(-0.342020143325662,0.,-0.939692620785911));
#15998=DIRECTION('ref_axis',(-0.939692620785911,0.,0.342020143325662));
#15999=DIRECTION('',(0.939692620785911,0.,-0.342020143325662));
#16000=DIRECTION('',(-0.939692620785911,0.,0.342020143325662));
#16001=DIRECTION('',(0.,1.,0.));
#16002=DIRECTION('center_axis',(-1.,0.,0.));
#16003=DIRECTION('ref_axis',(0.,0.,1.));
#16004=DIRECTION('',(0.,0.,-1.));
#16005=DIRECTION('',(0.,0.,1.));
#16006=DIRECTION('',(0.,1.,0.));
#16007=DIRECTION('center_axis',(-0.342020143325668,0.,0.939692620785909));
#16008=DIRECTION('ref_axis',(0.939692620785909,0.,0.342020143325668));
#16009=DIRECTION('',(-0.939692620785909,0.,-0.342020143325668));
#16010=DIRECTION('',(0.939692620785909,0.,0.342020143325668));
#16011=DIRECTION('',(0.,1.,0.));
#16012=DIRECTION('center_axis',(-1.,0.,0.));
#16013=DIRECTION('ref_axis',(0.,0.,1.));
#16014=DIRECTION('',(0.,0.,-1.));
#16015=DIRECTION('',(0.,0.,1.));
#16016=DIRECTION('',(0.,1.,0.));
#16017=DIRECTION('center_axis',(-0.342020143325668,0.,-0.939692620785909));
#16018=DIRECTION('ref_axis',(-0.939692620785909,0.,0.342020143325668));
#16019=DIRECTION('',(0.939692620785909,0.,-0.342020143325668));
#16020=DIRECTION('',(-0.939692620785909,0.,0.342020143325668));
#16021=DIRECTION('',(0.,1.,0.));
#16022=DIRECTION('center_axis',(-1.,0.,0.));
#16023=DIRECTION('ref_axis',(0.,0.,1.));
#16024=DIRECTION('',(0.,0.,-1.));
#16025=DIRECTION('',(0.,0.,1.));
#16026=DIRECTION('',(0.,1.,0.));
#16027=DIRECTION('center_axis',(-0.342020143325668,0.,0.939692620785909));
#16028=DIRECTION('ref_axis',(0.939692620785909,0.,0.342020143325668));
#16029=DIRECTION('',(-0.939692620785909,0.,-0.342020143325668));
#16030=DIRECTION('',(0.939692620785909,0.,0.342020143325668));
#16031=DIRECTION('',(0.,1.,0.));
#16032=DIRECTION('center_axis',(-1.,0.,0.));
#16033=DIRECTION('ref_axis',(0.,0.,1.));
#16034=DIRECTION('',(0.,0.,-1.));
#16035=DIRECTION('',(0.,0.,1.));
#16036=DIRECTION('',(0.,1.,0.));
#16037=DIRECTION('center_axis',(-0.342020143325668,0.,-0.939692620785909));
#16038=DIRECTION('ref_axis',(-0.939692620785909,0.,0.342020143325668));
#16039=DIRECTION('',(0.939692620785909,0.,-0.342020143325668));
#16040=DIRECTION('',(-0.939692620785909,0.,0.342020143325668));
#16041=DIRECTION('',(0.,1.,0.));
#16042=DIRECTION('center_axis',(-1.,0.,0.));
#16043=DIRECTION('ref_axis',(0.,0.,1.));
#16044=DIRECTION('',(0.,0.,-1.));
#16045=DIRECTION('',(0.,0.,1.));
#16046=DIRECTION('',(0.,1.,0.));
#16047=DIRECTION('center_axis',(-0.342020143325668,0.,0.939692620785909));
#16048=DIRECTION('ref_axis',(0.939692620785909,0.,0.342020143325668));
#16049=DIRECTION('',(-0.939692620785909,0.,-0.342020143325668));
#16050=DIRECTION('',(0.939692620785909,0.,0.342020143325668));
#16051=DIRECTION('',(0.,1.,0.));
#16052=DIRECTION('center_axis',(-1.,0.,0.));
#16053=DIRECTION('ref_axis',(0.,0.,1.));
#16054=DIRECTION('',(0.,0.,-1.));
#16055=DIRECTION('',(0.,0.,1.));
#16056=DIRECTION('',(0.,1.,0.));
#16057=DIRECTION('center_axis',(-0.342020143325662,0.,-0.939692620785911));
#16058=DIRECTION('ref_axis',(-0.939692620785911,0.,0.342020143325662));
#16059=DIRECTION('',(0.939692620785911,0.,-0.342020143325662));
#16060=DIRECTION('',(-0.939692620785911,0.,0.342020143325662));
#16061=DIRECTION('',(0.,1.,0.));
#16062=DIRECTION('center_axis',(-1.,0.,0.));
#16063=DIRECTION('ref_axis',(0.,0.,1.));
#16064=DIRECTION('',(0.,0.,-1.));
#16065=DIRECTION('',(0.,0.,1.));
#16066=DIRECTION('',(0.,1.,0.));
#16067=DIRECTION('center_axis',(-0.342020143325668,0.,0.939692620785909));
#16068=DIRECTION('ref_axis',(0.939692620785909,0.,0.342020143325668));
#16069=DIRECTION('',(-0.939692620785909,0.,-0.342020143325668));
#16070=DIRECTION('',(0.939692620785909,0.,0.342020143325668));
#16071=DIRECTION('',(0.,1.,0.));
#16072=DIRECTION('center_axis',(-1.,0.,0.));
#16073=DIRECTION('ref_axis',(0.,0.,1.));
#16074=DIRECTION('',(0.,0.,-1.));
#16075=DIRECTION('',(0.,0.,1.));
#16076=DIRECTION('',(0.,1.,0.));
#16077=DIRECTION('center_axis',(-0.342020143325668,0.,-0.939692620785909));
#16078=DIRECTION('ref_axis',(-0.939692620785909,0.,0.342020143325668));
#16079=DIRECTION('',(0.939692620785909,0.,-0.342020143325668));
#16080=DIRECTION('',(-0.939692620785909,0.,0.342020143325668));
#16081=DIRECTION('',(0.,1.,0.));
#16082=DIRECTION('center_axis',(-1.,0.,0.));
#16083=DIRECTION('ref_axis',(0.,0.,1.));
#16084=DIRECTION('',(0.,0.,-1.));
#16085=DIRECTION('',(0.,0.,1.));
#16086=DIRECTION('',(0.,1.,0.));
#16087=DIRECTION('center_axis',(-0.342020143325662,0.,0.939692620785911));
#16088=DIRECTION('ref_axis',(0.939692620785911,0.,0.342020143325662));
#16089=DIRECTION('',(-0.939692620785911,0.,-0.342020143325662));
#16090=DIRECTION('',(0.939692620785911,0.,0.342020143325662));
#16091=DIRECTION('',(0.,1.,0.));
#16092=DIRECTION('center_axis',(-1.,0.,0.));
#16093=DIRECTION('ref_axis',(0.,0.,1.));
#16094=DIRECTION('',(0.,0.,-1.));
#16095=DIRECTION('',(0.,0.,1.));
#16096=DIRECTION('',(0.,1.,0.));
#16097=DIRECTION('center_axis',(-0.342020143325668,0.,-0.939692620785909));
#16098=DIRECTION('ref_axis',(-0.939692620785909,0.,0.342020143325668));
#16099=DIRECTION('',(0.939692620785909,0.,-0.342020143325668));
#16100=DIRECTION('',(-0.939692620785909,0.,0.342020143325668));
#16101=DIRECTION('',(0.,1.,0.));
#16102=DIRECTION('center_axis',(-1.,0.,0.));
#16103=DIRECTION('ref_axis',(0.,0.,1.));
#16104=DIRECTION('',(0.,0.,-1.));
#16105=DIRECTION('',(0.,0.,1.));
#16106=DIRECTION('',(0.,1.,0.));
#16107=DIRECTION('center_axis',(-0.342020143325668,0.,0.939692620785909));
#16108=DIRECTION('ref_axis',(0.939692620785909,0.,0.342020143325668));
#16109=DIRECTION('',(-0.939692620785909,0.,-0.342020143325668));
#16110=DIRECTION('',(0.939692620785909,0.,0.342020143325668));
#16111=DIRECTION('',(0.,1.,0.));
#16112=DIRECTION('center_axis',(-1.,0.,0.));
#16113=DIRECTION('ref_axis',(0.,0.,1.));
#16114=DIRECTION('',(0.,0.,-1.));
#16115=DIRECTION('',(0.,0.,1.));
#16116=DIRECTION('',(0.,1.,0.));
#16117=DIRECTION('center_axis',(-0.342020143325668,0.,-0.939692620785909));
#16118=DIRECTION('ref_axis',(-0.939692620785909,0.,0.342020143325668));
#16119=DIRECTION('',(0.939692620785909,0.,-0.342020143325668));
#16120=DIRECTION('',(-0.939692620785909,0.,0.342020143325668));
#16121=DIRECTION('',(0.,1.,0.));
#16122=DIRECTION('center_axis',(-1.,0.,0.));
#16123=DIRECTION('ref_axis',(0.,0.,1.));
#16124=DIRECTION('',(0.,0.,-1.));
#16125=DIRECTION('',(0.,0.,1.));
#16126=DIRECTION('',(0.,1.,0.));
#16127=DIRECTION('center_axis',(-0.342020143325668,0.,0.939692620785909));
#16128=DIRECTION('ref_axis',(0.939692620785909,0.,0.342020143325668));
#16129=DIRECTION('',(-0.939692620785909,0.,-0.342020143325668));
#16130=DIRECTION('',(0.939692620785909,0.,0.342020143325668));
#16131=DIRECTION('',(0.,1.,0.));
#16132=DIRECTION('center_axis',(-1.,0.,0.));
#16133=DIRECTION('ref_axis',(0.,0.,1.));
#16134=DIRECTION('',(0.,0.,-1.));
#16135=DIRECTION('',(0.,0.,1.));
#16136=DIRECTION('',(0.,1.,0.));
#16137=DIRECTION('center_axis',(-0.342020143325662,0.,-0.939692620785911));
#16138=DIRECTION('ref_axis',(-0.939692620785911,0.,0.342020143325662));
#16139=DIRECTION('',(0.939692620785911,0.,-0.342020143325662));
#16140=DIRECTION('',(-0.939692620785911,0.,0.342020143325662));
#16141=DIRECTION('',(0.,1.,0.));
#16142=DIRECTION('center_axis',(-1.,0.,0.));
#16143=DIRECTION('ref_axis',(0.,0.,1.));
#16144=DIRECTION('',(0.,0.,-1.));
#16145=DIRECTION('',(0.,0.,1.));
#16146=DIRECTION('',(0.,1.,0.));
#16147=DIRECTION('center_axis',(-0.342020143325668,0.,0.939692620785909));
#16148=DIRECTION('ref_axis',(0.939692620785909,0.,0.342020143325668));
#16149=DIRECTION('',(-0.939692620785909,0.,-0.342020143325668));
#16150=DIRECTION('',(0.939692620785909,0.,0.342020143325668));
#16151=DIRECTION('',(0.,1.,0.));
#16152=DIRECTION('center_axis',(-1.,0.,0.));
#16153=DIRECTION('ref_axis',(0.,0.,1.));
#16154=DIRECTION('',(0.,0.,-1.));
#16155=DIRECTION('',(0.,0.,1.));
#16156=DIRECTION('',(0.,1.,0.));
#16157=DIRECTION('center_axis',(-0.342020143325668,0.,-0.939692620785909));
#16158=DIRECTION('ref_axis',(-0.939692620785909,0.,0.342020143325668));
#16159=DIRECTION('',(0.939692620785909,0.,-0.342020143325668));
#16160=DIRECTION('',(-0.939692620785909,0.,0.342020143325668));
#16161=DIRECTION('',(0.,1.,0.));
#16162=DIRECTION('center_axis',(-1.,0.,0.));
#16163=DIRECTION('ref_axis',(0.,0.,1.));
#16164=DIRECTION('',(0.,0.,-1.));
#16165=DIRECTION('',(0.,0.,1.));
#16166=DIRECTION('',(0.,1.,0.));
#16167=DIRECTION('center_axis',(-0.342020143325668,0.,0.939692620785909));
#16168=DIRECTION('ref_axis',(0.939692620785909,0.,0.342020143325668));
#16169=DIRECTION('',(-0.939692620785909,0.,-0.342020143325668));
#16170=DIRECTION('',(0.939692620785909,0.,0.342020143325668));
#16171=DIRECTION('',(0.,1.,0.));
#16172=DIRECTION('center_axis',(-1.,0.,0.));
#16173=DIRECTION('ref_axis',(0.,0.,1.));
#16174=DIRECTION('',(0.,0.,-1.));
#16175=DIRECTION('',(0.,0.,1.));
#16176=DIRECTION('',(0.,1.,0.));
#16177=DIRECTION('center_axis',(-0.342020143325668,0.,-0.939692620785909));
#16178=DIRECTION('ref_axis',(-0.939692620785909,0.,0.342020143325668));
#16179=DIRECTION('',(0.939692620785909,0.,-0.342020143325668));
#16180=DIRECTION('',(-0.939692620785909,0.,0.342020143325668));
#16181=DIRECTION('',(0.,1.,0.));
#16182=DIRECTION('center_axis',(-1.,0.,0.));
#16183=DIRECTION('ref_axis',(0.,0.,1.));
#16184=DIRECTION('',(0.,0.,-1.));
#16185=DIRECTION('',(0.,0.,1.));
#16186=DIRECTION('',(0.,1.,0.));
#16187=DIRECTION('center_axis',(-0.342020143325668,0.,0.939692620785909));
#16188=DIRECTION('ref_axis',(0.939692620785909,0.,0.342020143325668));
#16189=DIRECTION('',(-0.939692620785909,0.,-0.342020143325668));
#16190=DIRECTION('',(0.939692620785909,0.,0.342020143325668));
#16191=DIRECTION('',(0.,1.,0.));
#16192=DIRECTION('center_axis',(-1.,0.,0.));
#16193=DIRECTION('ref_axis',(0.,0.,1.));
#16194=DIRECTION('',(0.,0.,-1.));
#16195=DIRECTION('',(0.,0.,1.));
#16196=DIRECTION('',(0.,1.,0.));
#16197=DIRECTION('center_axis',(-0.342020143325668,0.,-0.939692620785909));
#16198=DIRECTION('ref_axis',(-0.939692620785909,0.,0.342020143325668));
#16199=DIRECTION('',(0.939692620785909,0.,-0.342020143325668));
#16200=DIRECTION('',(-0.939692620785909,0.,0.342020143325668));
#16201=DIRECTION('',(0.,1.,0.));
#16202=DIRECTION('center_axis',(-1.,0.,0.));
#16203=DIRECTION('ref_axis',(0.,0.,1.));
#16204=DIRECTION('',(0.,0.,-1.));
#16205=DIRECTION('',(0.,0.,1.));
#16206=DIRECTION('',(0.,1.,0.));
#16207=DIRECTION('center_axis',(-0.342020143325668,0.,0.939692620785909));
#16208=DIRECTION('ref_axis',(0.939692620785909,0.,0.342020143325668));
#16209=DIRECTION('',(-0.939692620785909,0.,-0.342020143325668));
#16210=DIRECTION('',(0.939692620785909,0.,0.342020143325668));
#16211=DIRECTION('',(0.,1.,0.));
#16212=DIRECTION('center_axis',(-1.,0.,0.));
#16213=DIRECTION('ref_axis',(0.,0.,1.));
#16214=DIRECTION('',(0.,0.,-1.));
#16215=DIRECTION('',(0.,0.,1.));
#16216=DIRECTION('',(0.,1.,0.));
#16217=DIRECTION('center_axis',(-0.342020143325662,0.,-0.939692620785911));
#16218=DIRECTION('ref_axis',(-0.939692620785911,0.,0.342020143325662));
#16219=DIRECTION('',(0.939692620785911,0.,-0.342020143325662));
#16220=DIRECTION('',(-0.939692620785911,0.,0.342020143325662));
#16221=DIRECTION('',(0.,1.,0.));
#16222=DIRECTION('center_axis',(-1.,0.,0.));
#16223=DIRECTION('ref_axis',(0.,0.,1.));
#16224=DIRECTION('',(0.,0.,-1.));
#16225=DIRECTION('',(0.,0.,1.));
#16226=DIRECTION('',(0.,1.,0.));
#16227=DIRECTION('center_axis',(-0.342020143325668,0.,0.939692620785909));
#16228=DIRECTION('ref_axis',(0.939692620785909,0.,0.342020143325668));
#16229=DIRECTION('',(-0.939692620785909,0.,-0.342020143325668));
#16230=DIRECTION('',(0.939692620785909,0.,0.342020143325668));
#16231=DIRECTION('',(0.,1.,0.));
#16232=DIRECTION('center_axis',(-1.,0.,0.));
#16233=DIRECTION('ref_axis',(0.,0.,1.));
#16234=DIRECTION('',(0.,0.,-1.));
#16235=DIRECTION('',(0.,0.,1.));
#16236=DIRECTION('',(0.,1.,0.));
#16237=DIRECTION('center_axis',(-0.342020143325668,0.,-0.939692620785909));
#16238=DIRECTION('ref_axis',(-0.939692620785909,0.,0.342020143325668));
#16239=DIRECTION('',(0.939692620785909,0.,-0.342020143325668));
#16240=DIRECTION('',(-0.939692620785909,0.,0.342020143325668));
#16241=DIRECTION('',(0.,1.,0.));
#16242=DIRECTION('center_axis',(-1.,0.,0.));
#16243=DIRECTION('ref_axis',(0.,0.,1.));
#16244=DIRECTION('',(0.,0.,-1.));
#16245=DIRECTION('',(0.,0.,1.));
#16246=DIRECTION('',(0.,1.,0.));
#16247=DIRECTION('center_axis',(-0.342020143325662,0.,0.939692620785911));
#16248=DIRECTION('ref_axis',(0.939692620785911,0.,0.342020143325662));
#16249=DIRECTION('',(-0.939692620785911,0.,-0.342020143325662));
#16250=DIRECTION('',(0.939692620785911,0.,0.342020143325662));
#16251=DIRECTION('',(0.,1.,0.));
#16252=DIRECTION('center_axis',(-1.,0.,0.));
#16253=DIRECTION('ref_axis',(0.,0.,1.));
#16254=DIRECTION('',(0.,0.,-1.));
#16255=DIRECTION('',(0.,0.,1.));
#16256=DIRECTION('',(0.,1.,0.));
#16257=DIRECTION('center_axis',(-0.342020143325668,0.,-0.939692620785909));
#16258=DIRECTION('ref_axis',(-0.939692620785909,0.,0.342020143325668));
#16259=DIRECTION('',(0.939692620785909,0.,-0.342020143325668));
#16260=DIRECTION('',(-0.939692620785909,0.,0.342020143325668));
#16261=DIRECTION('',(0.,1.,0.));
#16262=DIRECTION('center_axis',(-1.,0.,0.));
#16263=DIRECTION('ref_axis',(0.,0.,1.));
#16264=DIRECTION('',(0.,0.,-1.));
#16265=DIRECTION('',(0.,0.,1.));
#16266=DIRECTION('',(0.,1.,0.));
#16267=DIRECTION('center_axis',(-0.342020143325668,0.,0.939692620785909));
#16268=DIRECTION('ref_axis',(0.939692620785909,0.,0.342020143325668));
#16269=DIRECTION('',(-0.939692620785909,0.,-0.342020143325668));
#16270=DIRECTION('',(0.939692620785909,0.,0.342020143325668));
#16271=DIRECTION('',(0.,1.,0.));
#16272=DIRECTION('center_axis',(-1.,0.,0.));
#16273=DIRECTION('ref_axis',(0.,0.,1.));
#16274=DIRECTION('',(0.,0.,-1.));
#16275=DIRECTION('',(0.,0.,1.));
#16276=DIRECTION('',(0.,1.,0.));
#16277=DIRECTION('center_axis',(-0.342020143325668,0.,-0.939692620785909));
#16278=DIRECTION('ref_axis',(-0.939692620785909,0.,0.342020143325668));
#16279=DIRECTION('',(0.939692620785909,0.,-0.342020143325668));
#16280=DIRECTION('',(-0.939692620785909,0.,0.342020143325668));
#16281=DIRECTION('',(0.,1.,0.));
#16282=DIRECTION('center_axis',(-1.,0.,0.));
#16283=DIRECTION('ref_axis',(0.,0.,1.));
#16284=DIRECTION('',(0.,0.,-1.));
#16285=DIRECTION('',(0.,0.,1.));
#16286=DIRECTION('',(0.,1.,0.));
#16287=DIRECTION('center_axis',(-0.342020143325668,0.,0.939692620785909));
#16288=DIRECTION('ref_axis',(0.939692620785909,0.,0.342020143325668));
#16289=DIRECTION('',(-0.939692620785909,0.,-0.342020143325668));
#16290=DIRECTION('',(0.939692620785909,0.,0.342020143325668));
#16291=DIRECTION('',(0.,1.,0.));
#16292=DIRECTION('center_axis',(-1.,0.,0.));
#16293=DIRECTION('ref_axis',(0.,0.,1.));
#16294=DIRECTION('',(0.,0.,-1.));
#16295=DIRECTION('',(0.,0.,1.));
#16296=DIRECTION('',(0.,1.,0.));
#16297=DIRECTION('center_axis',(-0.342020143325662,0.,-0.939692620785911));
#16298=DIRECTION('ref_axis',(-0.939692620785911,0.,0.342020143325662));
#16299=DIRECTION('',(0.939692620785911,0.,-0.342020143325662));
#16300=DIRECTION('',(-0.939692620785911,0.,0.342020143325662));
#16301=DIRECTION('',(0.,1.,0.));
#16302=DIRECTION('center_axis',(-1.,0.,0.));
#16303=DIRECTION('ref_axis',(0.,0.,1.));
#16304=DIRECTION('',(0.,0.,-1.));
#16305=DIRECTION('',(0.,0.,1.));
#16306=DIRECTION('',(0.,1.,0.));
#16307=DIRECTION('center_axis',(-0.342020143325668,0.,0.939692620785909));
#16308=DIRECTION('ref_axis',(0.939692620785909,0.,0.342020143325668));
#16309=DIRECTION('',(-0.939692620785909,0.,-0.342020143325668));
#16310=DIRECTION('',(0.939692620785909,0.,0.342020143325668));
#16311=DIRECTION('',(0.,1.,0.));
#16312=DIRECTION('center_axis',(-1.,0.,0.));
#16313=DIRECTION('ref_axis',(0.,0.,1.));
#16314=DIRECTION('',(0.,0.,-1.));
#16315=DIRECTION('',(0.,0.,1.));
#16316=DIRECTION('',(0.,1.,0.));
#16317=DIRECTION('center_axis',(-0.342020143325668,0.,-0.939692620785909));
#16318=DIRECTION('ref_axis',(-0.939692620785909,0.,0.342020143325668));
#16319=DIRECTION('',(0.939692620785909,0.,-0.342020143325668));
#16320=DIRECTION('',(-0.939692620785909,0.,0.342020143325668));
#16321=DIRECTION('',(0.,1.,0.));
#16322=DIRECTION('center_axis',(-1.,0.,0.));
#16323=DIRECTION('ref_axis',(0.,0.,1.));
#16324=DIRECTION('',(0.,0.,-1.));
#16325=DIRECTION('',(0.,0.,1.));
#16326=DIRECTION('',(0.,1.,0.));
#16327=DIRECTION('center_axis',(-0.342020143325668,0.,0.939692620785909));
#16328=DIRECTION('ref_axis',(0.939692620785909,0.,0.342020143325668));
#16329=DIRECTION('',(-0.939692620785909,0.,-0.342020143325668));
#16330=DIRECTION('',(0.939692620785909,0.,0.342020143325668));
#16331=DIRECTION('',(0.,1.,0.));
#16332=DIRECTION('center_axis',(-1.,0.,0.));
#16333=DIRECTION('ref_axis',(0.,0.,1.));
#16334=DIRECTION('',(0.,0.,-1.));
#16335=DIRECTION('',(0.,0.,1.));
#16336=DIRECTION('',(0.,1.,0.));
#16337=DIRECTION('center_axis',(-0.342020143325668,0.,-0.939692620785909));
#16338=DIRECTION('ref_axis',(-0.939692620785909,0.,0.342020143325668));
#16339=DIRECTION('',(0.939692620785909,0.,-0.342020143325668));
#16340=DIRECTION('',(-0.939692620785909,0.,0.342020143325668));
#16341=DIRECTION('',(0.,1.,0.));
#16342=DIRECTION('center_axis',(-1.,0.,0.));
#16343=DIRECTION('ref_axis',(0.,0.,1.));
#16344=DIRECTION('',(0.,0.,-1.));
#16345=DIRECTION('',(0.,0.,1.));
#16346=DIRECTION('',(0.,1.,0.));
#16347=DIRECTION('center_axis',(-0.342020143325668,0.,0.939692620785909));
#16348=DIRECTION('ref_axis',(0.939692620785909,0.,0.342020143325668));
#16349=DIRECTION('',(-0.939692620785909,0.,-0.342020143325668));
#16350=DIRECTION('',(0.939692620785909,0.,0.342020143325668));
#16351=DIRECTION('',(0.,1.,0.));
#16352=DIRECTION('center_axis',(-1.,0.,0.));
#16353=DIRECTION('ref_axis',(0.,0.,1.));
#16354=DIRECTION('',(0.,0.,-1.));
#16355=DIRECTION('',(0.,0.,1.));
#16356=DIRECTION('',(0.,1.,0.));
#16357=DIRECTION('center_axis',(-0.342020143325665,0.,-0.93969262078591));
#16358=DIRECTION('ref_axis',(-0.93969262078591,0.,0.342020143325665));
#16359=DIRECTION('',(0.93969262078591,0.,-0.342020143325665));
#16360=DIRECTION('',(-0.93969262078591,0.,0.342020143325665));
#16361=DIRECTION('',(0.,1.,0.));
#16362=DIRECTION('center_axis',(-1.,0.,0.));
#16363=DIRECTION('ref_axis',(0.,0.,1.));
#16364=DIRECTION('',(0.,0.,-1.));
#16365=DIRECTION('',(0.,0.,1.));
#16366=DIRECTION('',(0.,1.,0.));
#16367=DIRECTION('center_axis',(-0.342020143325668,0.,0.939692620785909));
#16368=DIRECTION('ref_axis',(0.939692620785909,0.,0.342020143325668));
#16369=DIRECTION('',(-0.939692620785909,0.,-0.342020143325668));
#16370=DIRECTION('',(0.939692620785909,0.,0.342020143325668));
#16371=DIRECTION('',(0.,1.,0.));
#16372=DIRECTION('center_axis',(-1.,0.,0.));
#16373=DIRECTION('ref_axis',(0.,0.,1.));
#16374=DIRECTION('',(0.,0.,-1.));
#16375=DIRECTION('',(0.,0.,1.));
#16376=DIRECTION('',(0.,1.,0.));
#16377=DIRECTION('center_axis',(-0.342020143325668,0.,-0.939692620785909));
#16378=DIRECTION('ref_axis',(-0.939692620785909,0.,0.342020143325668));
#16379=DIRECTION('',(0.939692620785909,0.,-0.342020143325668));
#16380=DIRECTION('',(-0.939692620785909,0.,0.342020143325668));
#16381=DIRECTION('',(0.,1.,0.));
#16382=DIRECTION('center_axis',(-1.,0.,0.));
#16383=DIRECTION('ref_axis',(0.,0.,1.));
#16384=DIRECTION('',(0.,0.,-1.));
#16385=DIRECTION('',(0.,0.,1.));
#16386=DIRECTION('',(0.,1.,0.));
#16387=DIRECTION('center_axis',(-0.342020143325665,0.,0.93969262078591));
#16388=DIRECTION('ref_axis',(0.93969262078591,0.,0.342020143325665));
#16389=DIRECTION('',(-0.93969262078591,0.,-0.342020143325665));
#16390=DIRECTION('',(0.93969262078591,0.,0.342020143325665));
#16391=DIRECTION('',(0.,1.,0.));
#16392=DIRECTION('center_axis',(-1.,0.,0.));
#16393=DIRECTION('ref_axis',(0.,0.,1.));
#16394=DIRECTION('',(0.,0.,-1.));
#16395=DIRECTION('',(0.,0.,1.));
#16396=DIRECTION('',(0.,1.,0.));
#16397=DIRECTION('center_axis',(-0.342020143325665,0.,-0.93969262078591));
#16398=DIRECTION('ref_axis',(-0.93969262078591,0.,0.342020143325665));
#16399=DIRECTION('',(0.93969262078591,0.,-0.342020143325665));
#16400=DIRECTION('',(-0.93969262078591,0.,0.342020143325665));
#16401=DIRECTION('',(0.,1.,0.));
#16402=DIRECTION('center_axis',(-1.,0.,0.));
#16403=DIRECTION('ref_axis',(0.,0.,1.));
#16404=DIRECTION('',(0.,0.,-1.));
#16405=DIRECTION('',(0.,0.,1.));
#16406=DIRECTION('',(0.,1.,0.));
#16407=DIRECTION('center_axis',(-0.342020143325668,0.,0.939692620785909));
#16408=DIRECTION('ref_axis',(0.939692620785909,0.,0.342020143325668));
#16409=DIRECTION('',(-0.939692620785909,0.,-0.342020143325668));
#16410=DIRECTION('',(0.939692620785909,0.,0.342020143325668));
#16411=DIRECTION('',(0.,1.,0.));
#16412=DIRECTION('center_axis',(-1.,0.,0.));
#16413=DIRECTION('ref_axis',(0.,0.,1.));
#16414=DIRECTION('',(0.,0.,-1.));
#16415=DIRECTION('',(0.,0.,1.));
#16416=DIRECTION('',(0.,1.,0.));
#16417=DIRECTION('center_axis',(-0.342020143325668,0.,-0.939692620785909));
#16418=DIRECTION('ref_axis',(-0.939692620785909,0.,0.342020143325668));
#16419=DIRECTION('',(0.939692620785909,0.,-0.342020143325668));
#16420=DIRECTION('',(-0.939692620785909,0.,0.342020143325668));
#16421=DIRECTION('',(0.,1.,0.));
#16422=DIRECTION('center_axis',(-1.,0.,0.));
#16423=DIRECTION('ref_axis',(0.,0.,1.));
#16424=DIRECTION('',(0.,0.,-1.));
#16425=DIRECTION('',(0.,0.,1.));
#16426=DIRECTION('',(0.,1.,0.));
#16427=DIRECTION('center_axis',(-0.342020143325668,0.,0.939692620785909));
#16428=DIRECTION('ref_axis',(0.939692620785909,0.,0.342020143325668));
#16429=DIRECTION('',(-0.939692620785909,0.,-0.342020143325668));
#16430=DIRECTION('',(0.939692620785909,0.,0.342020143325668));
#16431=DIRECTION('',(0.,1.,0.));
#16432=DIRECTION('center_axis',(-1.,0.,0.));
#16433=DIRECTION('ref_axis',(0.,0.,1.));
#16434=DIRECTION('',(0.,0.,-1.));
#16435=DIRECTION('',(0.,0.,1.));
#16436=DIRECTION('',(0.,1.,0.));
#16437=DIRECTION('center_axis',(-0.342020143325665,0.,-0.93969262078591));
#16438=DIRECTION('ref_axis',(-0.93969262078591,0.,0.342020143325665));
#16439=DIRECTION('',(0.93969262078591,0.,-0.342020143325665));
#16440=DIRECTION('',(-0.93969262078591,0.,0.342020143325665));
#16441=DIRECTION('',(0.,1.,0.));
#16442=DIRECTION('center_axis',(-1.,0.,0.));
#16443=DIRECTION('ref_axis',(0.,0.,1.));
#16444=DIRECTION('',(0.,0.,-1.));
#16445=DIRECTION('',(0.,0.,1.));
#16446=DIRECTION('',(0.,1.,0.));
#16447=DIRECTION('center_axis',(-0.342020143325668,0.,0.939692620785909));
#16448=DIRECTION('ref_axis',(0.939692620785909,0.,0.342020143325668));
#16449=DIRECTION('',(-0.939692620785909,0.,-0.342020143325668));
#16450=DIRECTION('',(0.939692620785909,0.,0.342020143325668));
#16451=DIRECTION('',(0.,1.,0.));
#16452=DIRECTION('center_axis',(-1.,0.,0.));
#16453=DIRECTION('ref_axis',(0.,0.,1.));
#16454=DIRECTION('',(0.,0.,-1.));
#16455=DIRECTION('',(0.,0.,1.));
#16456=DIRECTION('',(0.,1.,0.));
#16457=DIRECTION('center_axis',(-0.342020143325671,0.,-0.939692620785907));
#16458=DIRECTION('ref_axis',(-0.939692620785907,0.,0.342020143325671));
#16459=DIRECTION('',(0.939692620785907,0.,-0.342020143325671));
#16460=DIRECTION('',(-0.939692620785907,0.,0.342020143325671));
#16461=DIRECTION('',(0.,1.,0.));
#16462=DIRECTION('center_axis',(-1.,0.,0.));
#16463=DIRECTION('ref_axis',(0.,0.,1.));
#16464=DIRECTION('',(0.,0.,-1.));
#16465=DIRECTION('',(0.,0.,1.));
#16466=DIRECTION('',(0.,1.,0.));
#16467=DIRECTION('center_axis',(-0.342020143325668,0.,0.939692620785909));
#16468=DIRECTION('ref_axis',(0.939692620785909,0.,0.342020143325668));
#16469=DIRECTION('',(-0.939692620785909,0.,-0.342020143325668));
#16470=DIRECTION('',(0.939692620785909,0.,0.342020143325668));
#16471=DIRECTION('',(0.,1.,0.));
#16472=DIRECTION('center_axis',(-1.,0.,0.));
#16473=DIRECTION('ref_axis',(0.,0.,1.));
#16474=DIRECTION('',(0.,0.,-1.));
#16475=DIRECTION('',(0.,0.,1.));
#16476=DIRECTION('',(0.,1.,0.));
#16477=DIRECTION('center_axis',(-0.342020143325668,0.,-0.939692620785909));
#16478=DIRECTION('ref_axis',(-0.939692620785909,0.,0.342020143325668));
#16479=DIRECTION('',(0.939692620785909,0.,-0.342020143325668));
#16480=DIRECTION('',(-0.939692620785909,0.,0.342020143325668));
#16481=DIRECTION('',(0.,1.,0.));
#16482=DIRECTION('center_axis',(-1.,0.,0.));
#16483=DIRECTION('ref_axis',(0.,0.,1.));
#16484=DIRECTION('',(0.,0.,-1.));
#16485=DIRECTION('',(0.,0.,1.));
#16486=DIRECTION('',(0.,1.,0.));
#16487=DIRECTION('center_axis',(-0.342020143325668,0.,0.939692620785909));
#16488=DIRECTION('ref_axis',(0.939692620785909,0.,0.342020143325668));
#16489=DIRECTION('',(-0.939692620785909,0.,-0.342020143325668));
#16490=DIRECTION('',(0.939692620785909,0.,0.342020143325668));
#16491=DIRECTION('',(0.,1.,0.));
#16492=DIRECTION('center_axis',(-1.,0.,0.));
#16493=DIRECTION('ref_axis',(0.,0.,1.));
#16494=DIRECTION('',(0.,0.,-1.));
#16495=DIRECTION('',(0.,0.,1.));
#16496=DIRECTION('',(0.,1.,0.));
#16497=DIRECTION('center_axis',(-0.342020143325671,0.,-0.939692620785907));
#16498=DIRECTION('ref_axis',(-0.939692620785907,0.,0.342020143325671));
#16499=DIRECTION('',(0.939692620785907,0.,-0.342020143325671));
#16500=DIRECTION('',(-0.939692620785907,0.,0.342020143325671));
#16501=DIRECTION('',(0.,1.,0.));
#16502=DIRECTION('center_axis',(-1.,0.,0.));
#16503=DIRECTION('ref_axis',(0.,0.,1.));
#16504=DIRECTION('',(0.,0.,-1.));
#16505=DIRECTION('',(0.,0.,1.));
#16506=DIRECTION('center_axis',(0.,1.,0.));
#16507=DIRECTION('ref_axis',(0.,0.,1.));
#16508=DIRECTION('center_axis',(0.,1.,0.));
#16509=DIRECTION('ref_axis',(1.,0.,0.));
#16510=DIRECTION('center_axis',(0.,0.,1.));
#16511=DIRECTION('ref_axis',(1.,0.,0.));
#16512=DIRECTION('center_axis',(0.,0.,1.));
#16513=DIRECTION('ref_axis',(1.,0.,0.));
#16514=DIRECTION('',(0.,0.,-1.));
#16515=DIRECTION('',(0.,0.,-1.));
#16516=DIRECTION('center_axis',(0.,0.,1.));
#16517=DIRECTION('ref_axis',(1.,0.,0.));
#16518=DIRECTION('center_axis',(0.,0.,1.));
#16519=DIRECTION('ref_axis',(1.,0.,0.));
#16520=DIRECTION('center_axis',(0.,0.,1.));
#16521=DIRECTION('ref_axis',(1.,0.,0.));
#19315=CARTESIAN_POINT('',(0.,0.,0.));
#19316=CARTESIAN_POINT('Origin',(1.,0.,10.7));
#19317=CARTESIAN_POINT('',(0.575,-5.20474889637625E-17,10.8));
#19318=CARTESIAN_POINT('Origin',(1.,0.,10.8));
#19319=CARTESIAN_POINT('',(0.575,-5.20474889637625E-17,12.));
#19320=CARTESIAN_POINT('',(0.575,-5.20474889637625E-17,10.7));
#19321=CARTESIAN_POINT('Origin',(1.,0.,12.));
#19322=CARTESIAN_POINT('Origin',(1.,0.,12.));
#19323=CARTESIAN_POINT('Origin',(0.2,-1.,37.));
#19324=CARTESIAN_POINT('',(0.2,-0.6,37.));
#19325=CARTESIAN_POINT('',(0.2,-0.6,11.));
#19326=CARTESIAN_POINT('',(0.2,-0.6,10.8));
#19327=CARTESIAN_POINT('',(0.2,-1.,37.));
#19328=CARTESIAN_POINT('',(0.2,-1.,37.));
#19329=CARTESIAN_POINT('',(0.2,-1.,11.));
#19330=CARTESIAN_POINT('',(0.2,-1.,11.));
#19331=CARTESIAN_POINT('',(0.2,-1.,11.));
#19332=CARTESIAN_POINT('Origin',(0.2,-1.,37.));
#19333=CARTESIAN_POINT('',(0.2,0.6,11.));
#19334=CARTESIAN_POINT('',(0.2,0.6,37.));
#19335=CARTESIAN_POINT('',(0.2,0.6,10.8));
#19336=CARTESIAN_POINT('',(0.2,1.,11.));
#19337=CARTESIAN_POINT('',(0.2,-1.,11.));
#19338=CARTESIAN_POINT('',(0.2,1.,37.));
#19339=CARTESIAN_POINT('',(0.2,1.,11.));
#19340=CARTESIAN_POINT('',(0.2,-1.,37.));
#19341=CARTESIAN_POINT('Origin',(0.2,-1.,11.));
#19342=CARTESIAN_POINT('',(0.,-1.22464679914735E-16,11.));
#19343=CARTESIAN_POINT('Origin',(1.,0.,11.));
#19344=CARTESIAN_POINT('',(-1.,-1.,11.));
#19345=CARTESIAN_POINT('',(-1.,-1.,11.));
#19346=CARTESIAN_POINT('',(-1.,1.,11.));
#19347=CARTESIAN_POINT('',(-1.,-1.,11.));
#19348=CARTESIAN_POINT('',(-1.,1.,11.));
#19349=CARTESIAN_POINT('Origin',(1.,0.,11.));
#19350=CARTESIAN_POINT('Origin',(-1.,-1.,37.));
#19351=CARTESIAN_POINT('',(0.,-1.22464679914735E-16,37.));
#19352=CARTESIAN_POINT('Origin',(1.,0.,37.));
#19353=CARTESIAN_POINT('',(-1.,1.,37.));
#19354=CARTESIAN_POINT('',(0.2,1.,37.));
#19355=CARTESIAN_POINT('',(-1.,-1.,37.));
#19356=CARTESIAN_POINT('',(-1.,-1.,37.));
#19357=CARTESIAN_POINT('',(0.2,-1.,37.));
#19358=CARTESIAN_POINT('Origin',(1.,0.,37.));
#19359=CARTESIAN_POINT('Origin',(-1.,-1.,36.269194724554));
#19360=CARTESIAN_POINT('',(-1.,-1.,36.269194724554));
#19361=CARTESIAN_POINT('',(-1.,-1.,37.));
#19362=CARTESIAN_POINT('',(-1.,1.,36.269194724554));
#19363=CARTESIAN_POINT('',(-1.,1.,37.));
#19364=CARTESIAN_POINT('',(-1.,-1.,36.269194724554));
#19365=CARTESIAN_POINT('Origin',(-1.45,-1.,36.1054081191342));
#19366=CARTESIAN_POINT('',(-1.45,-1.,36.1054081191342));
#19367=CARTESIAN_POINT('',(-1.,-1.,36.269194724554));
#19368=CARTESIAN_POINT('',(-1.45,1.,36.1054081191342));
#19369=CARTESIAN_POINT('',(-1.,1.,36.269194724554));
#19370=CARTESIAN_POINT('',(-1.45,-1.,36.1054081191342));
#19371=CARTESIAN_POINT('Origin',(-1.45,-1.,35.9388369474817));
#19372=CARTESIAN_POINT('',(-1.45,-1.,35.9388369474817));
#19373=CARTESIAN_POINT('',(-1.45,-1.,36.1054081191342));
#19374=CARTESIAN_POINT('',(-1.45,1.,35.9388369474817));
#19375=CARTESIAN_POINT('',(-1.45,1.,36.1054081191342));
#19376=CARTESIAN_POINT('',(-1.45,-1.,35.9388369474817));
#19377=CARTESIAN_POINT('Origin',(-1.,-1.,35.7750503420619));
#19378=CARTESIAN_POINT('',(-1.,-1.,35.7750503420619));
#19379=CARTESIAN_POINT('',(-1.45,-1.,35.9388369474817));
#19380=CARTESIAN_POINT('',(-1.,1.,35.7750503420619));
#19381=CARTESIAN_POINT('',(-1.45,1.,35.9388369474817));
#19382=CARTESIAN_POINT('',(-1.,-1.,35.7750503420619));
#19383=CARTESIAN_POINT('Origin',(-1.,-1.,35.640876193836));
#19384=CARTESIAN_POINT('',(-1.,-1.,35.640876193836));
#19385=CARTESIAN_POINT('',(-1.,-1.,35.7750503420619));
#19386=CARTESIAN_POINT('',(-1.,1.,35.640876193836));
#19387=CARTESIAN_POINT('',(-1.,1.,35.7750503420619));
#19388=CARTESIAN_POINT('',(-1.,-1.,35.640876193836));
#19389=CARTESIAN_POINT('Origin',(-1.45,-1.,35.4770895884162));
#19390=CARTESIAN_POINT('',(-1.45,-1.,35.4770895884162));
#19391=CARTESIAN_POINT('',(-1.,-1.,35.640876193836));
#19392=CARTESIAN_POINT('',(-1.45,1.,35.4770895884162));
#19393=CARTESIAN_POINT('',(-1.,1.,35.640876193836));
#19394=CARTESIAN_POINT('',(-1.45,-1.,35.4770895884162));
#19395=CARTESIAN_POINT('Origin',(-1.45,-1.,35.3105184167637));
#19396=CARTESIAN_POINT('',(-1.45,-1.,35.3105184167637));
#19397=CARTESIAN_POINT('',(-1.45,-1.,35.4770895884162));
#19398=CARTESIAN_POINT('',(-1.45,1.,35.3105184167637));
#19399=CARTESIAN_POINT('',(-1.45,1.,35.4770895884162));
#19400=CARTESIAN_POINT('',(-1.45,-1.,35.3105184167637));
#19401=CARTESIAN_POINT('Origin',(-1.,-1.,35.1467318113439));
#19402=CARTESIAN_POINT('',(-1.,-1.,35.1467318113439));
#19403=CARTESIAN_POINT('',(-1.45,-1.,35.3105184167637));
#19404=CARTESIAN_POINT('',(-1.,1.,35.1467318113439));
#19405=CARTESIAN_POINT('',(-1.45,1.,35.3105184167637));
#19406=CARTESIAN_POINT('',(-1.,-1.,35.1467318113439));
#19407=CARTESIAN_POINT('Origin',(-1.,-1.,35.0125576631181));
#19408=CARTESIAN_POINT('',(-1.,-1.,35.0125576631181));
#19409=CARTESIAN_POINT('',(-1.,-1.,35.1467318113439));
#19410=CARTESIAN_POINT('',(-1.,1.,35.0125576631181));
#19411=CARTESIAN_POINT('',(-1.,1.,35.1467318113439));
#19412=CARTESIAN_POINT('',(-1.,-1.,35.0125576631181));
#19413=CARTESIAN_POINT('Origin',(-1.45,-1.,34.8487710576983));
#19414=CARTESIAN_POINT('',(-1.45,-1.,34.8487710576983));
#19415=CARTESIAN_POINT('',(-1.,-1.,35.0125576631181));
#19416=CARTESIAN_POINT('',(-1.45,1.,34.8487710576983));
#19417=CARTESIAN_POINT('',(-1.,1.,35.0125576631181));
#19418=CARTESIAN_POINT('',(-1.45,-1.,34.8487710576983));
#19419=CARTESIAN_POINT('Origin',(-1.45,-1.,34.6821998860458));
#19420=CARTESIAN_POINT('',(-1.45,-1.,34.6821998860458));
#19421=CARTESIAN_POINT('',(-1.45,-1.,34.8487710576983));
#19422=CARTESIAN_POINT('',(-1.45,1.,34.6821998860458));
#19423=CARTESIAN_POINT('',(-1.45,1.,34.8487710576983));
#19424=CARTESIAN_POINT('',(-1.45,-1.,34.6821998860458));
#19425=CARTESIAN_POINT('Origin',(-1.,-1.,34.518413280626));
#19426=CARTESIAN_POINT('',(-1.,-1.,34.518413280626));
#19427=CARTESIAN_POINT('',(-1.45,-1.,34.6821998860458));
#19428=CARTESIAN_POINT('',(-1.,1.,34.518413280626));
#19429=CARTESIAN_POINT('',(-1.45,1.,34.6821998860458));
#19430=CARTESIAN_POINT('',(-1.,-1.,34.518413280626));
#19431=CARTESIAN_POINT('Origin',(-1.,-1.,34.3842391324001));
#19432=CARTESIAN_POINT('',(-1.,-1.,34.3842391324001));
#19433=CARTESIAN_POINT('',(-1.,-1.,34.518413280626));
#19434=CARTESIAN_POINT('',(-1.,1.,34.3842391324001));
#19435=CARTESIAN_POINT('',(-1.,1.,34.518413280626));
#19436=CARTESIAN_POINT('',(-1.,-1.,34.3842391324001));
#19437=CARTESIAN_POINT('Origin',(-1.45,-1.,34.2204525269803));
#19438=CARTESIAN_POINT('',(-1.45,-1.,34.2204525269803));
#19439=CARTESIAN_POINT('',(-1.,-1.,34.3842391324001));
#19440=CARTESIAN_POINT('',(-1.45,1.,34.2204525269803));
#19441=CARTESIAN_POINT('',(-1.,1.,34.3842391324001));
#19442=CARTESIAN_POINT('',(-1.45,-1.,34.2204525269803));
#19443=CARTESIAN_POINT('Origin',(-1.45,-1.,34.0538813553278));
#19444=CARTESIAN_POINT('',(-1.45,-1.,34.0538813553278));
#19445=CARTESIAN_POINT('',(-1.45,-1.,34.2204525269803));
#19446=CARTESIAN_POINT('',(-1.45,1.,34.0538813553278));
#19447=CARTESIAN_POINT('',(-1.45,1.,34.2204525269803));
#19448=CARTESIAN_POINT('',(-1.45,-1.,34.0538813553278));
#19449=CARTESIAN_POINT('Origin',(-1.,-1.,33.890094749908));
#19450=CARTESIAN_POINT('',(-1.,-1.,33.890094749908));
#19451=CARTESIAN_POINT('',(-1.45,-1.,34.0538813553278));
#19452=CARTESIAN_POINT('',(-1.,1.,33.890094749908));
#19453=CARTESIAN_POINT('',(-1.45,1.,34.0538813553278));
#19454=CARTESIAN_POINT('',(-1.,-1.,33.890094749908));
#19455=CARTESIAN_POINT('Origin',(-1.,-1.,33.7559206016821));
#19456=CARTESIAN_POINT('',(-1.,-1.,33.7559206016821));
#19457=CARTESIAN_POINT('',(-1.,-1.,33.890094749908));
#19458=CARTESIAN_POINT('',(-1.,1.,33.7559206016821));
#19459=CARTESIAN_POINT('',(-1.,1.,33.890094749908));
#19460=CARTESIAN_POINT('',(-1.,-1.,33.7559206016821));
#19461=CARTESIAN_POINT('Origin',(-1.45,-1.,33.5921339962624));
#19462=CARTESIAN_POINT('',(-1.45,-1.,33.5921339962624));
#19463=CARTESIAN_POINT('',(-1.,-1.,33.7559206016821));
#19464=CARTESIAN_POINT('',(-1.45,1.,33.5921339962624));
#19465=CARTESIAN_POINT('',(-1.,1.,33.7559206016821));
#19466=CARTESIAN_POINT('',(-1.45,-1.,33.5921339962624));
#19467=CARTESIAN_POINT('Origin',(-1.45,-1.,33.4255628246099));
#19468=CARTESIAN_POINT('',(-1.45,-1.,33.4255628246099));
#19469=CARTESIAN_POINT('',(-1.45,-1.,33.5921339962624));
#19470=CARTESIAN_POINT('',(-1.45,1.,33.4255628246099));
#19471=CARTESIAN_POINT('',(-1.45,1.,33.5921339962624));
#19472=CARTESIAN_POINT('',(-1.45,-1.,33.4255628246099));
#19473=CARTESIAN_POINT('Origin',(-1.,-1.,33.2617762191901));
#19474=CARTESIAN_POINT('',(-1.,-1.,33.2617762191901));
#19475=CARTESIAN_POINT('',(-1.45,-1.,33.4255628246099));
#19476=CARTESIAN_POINT('',(-1.,1.,33.2617762191901));
#19477=CARTESIAN_POINT('',(-1.45,1.,33.4255628246099));
#19478=CARTESIAN_POINT('',(-1.,-1.,33.2617762191901));
#19479=CARTESIAN_POINT('Origin',(-1.,-1.,33.1276020709642));
#19480=CARTESIAN_POINT('',(-1.,-1.,33.1276020709642));
#19481=CARTESIAN_POINT('',(-1.,-1.,33.2617762191901));
#19482=CARTESIAN_POINT('',(-1.,1.,33.1276020709642));
#19483=CARTESIAN_POINT('',(-1.,1.,33.2617762191901));
#19484=CARTESIAN_POINT('',(-1.,-1.,33.1276020709642));
#19485=CARTESIAN_POINT('Origin',(-1.45,-1.,32.9638154655444));
#19486=CARTESIAN_POINT('',(-1.45,-1.,32.9638154655444));
#19487=CARTESIAN_POINT('',(-1.,-1.,33.1276020709642));
#19488=CARTESIAN_POINT('',(-1.45,1.,32.9638154655444));
#19489=CARTESIAN_POINT('',(-1.,1.,33.1276020709642));
#19490=CARTESIAN_POINT('',(-1.45,-1.,32.9638154655444));
#19491=CARTESIAN_POINT('Origin',(-1.45,-1.,32.7972442938919));
#19492=CARTESIAN_POINT('',(-1.45,-1.,32.7972442938919));
#19493=CARTESIAN_POINT('',(-1.45,-1.,32.9638154655444));
#19494=CARTESIAN_POINT('',(-1.45,1.,32.7972442938919));
#19495=CARTESIAN_POINT('',(-1.45,1.,32.9638154655444));
#19496=CARTESIAN_POINT('',(-1.45,-1.,32.7972442938919));
#19497=CARTESIAN_POINT('Origin',(-1.,-1.,32.6334576884721));
#19498=CARTESIAN_POINT('',(-1.,-1.,32.6334576884721));
#19499=CARTESIAN_POINT('',(-1.45,-1.,32.7972442938919));
#19500=CARTESIAN_POINT('',(-1.,1.,32.6334576884721));
#19501=CARTESIAN_POINT('',(-1.45,1.,32.7972442938919));
#19502=CARTESIAN_POINT('',(-1.,-1.,32.6334576884721));
#19503=CARTESIAN_POINT('Origin',(-1.,-1.,32.4992835402462));
#19504=CARTESIAN_POINT('',(-1.,-1.,32.4992835402462));
#19505=CARTESIAN_POINT('',(-1.,-1.,32.6334576884721));
#19506=CARTESIAN_POINT('',(-1.,1.,32.4992835402462));
#19507=CARTESIAN_POINT('',(-1.,1.,32.6334576884721));
#19508=CARTESIAN_POINT('',(-1.,-1.,32.4992835402462));
#19509=CARTESIAN_POINT('Origin',(-1.45,-1.,32.3354969348264));
#19510=CARTESIAN_POINT('',(-1.45,-1.,32.3354969348264));
#19511=CARTESIAN_POINT('',(-1.,-1.,32.4992835402462));
#19512=CARTESIAN_POINT('',(-1.45,1.,32.3354969348264));
#19513=CARTESIAN_POINT('',(-1.,1.,32.4992835402462));
#19514=CARTESIAN_POINT('',(-1.45,-1.,32.3354969348264));
#19515=CARTESIAN_POINT('Origin',(-1.45,-1.,32.1689257631739));
#19516=CARTESIAN_POINT('',(-1.45,-1.,32.1689257631739));
#19517=CARTESIAN_POINT('',(-1.45,-1.,32.3354969348264));
#19518=CARTESIAN_POINT('',(-1.45,1.,32.1689257631739));
#19519=CARTESIAN_POINT('',(-1.45,1.,32.3354969348264));
#19520=CARTESIAN_POINT('',(-1.45,-1.,32.1689257631739));
#19521=CARTESIAN_POINT('Origin',(-1.,-1.,32.0051391577542));
#19522=CARTESIAN_POINT('',(-1.,-1.,32.0051391577542));
#19523=CARTESIAN_POINT('',(-1.45,-1.,32.1689257631739));
#19524=CARTESIAN_POINT('',(-1.,1.,32.0051391577542));
#19525=CARTESIAN_POINT('',(-1.45,1.,32.1689257631739));
#19526=CARTESIAN_POINT('',(-1.,-1.,32.0051391577542));
#19527=CARTESIAN_POINT('Origin',(-1.,-1.,31.8709650095283));
#19528=CARTESIAN_POINT('',(-1.,-1.,31.8709650095283));
#19529=CARTESIAN_POINT('',(-1.,-1.,32.0051391577542));
#19530=CARTESIAN_POINT('',(-1.,1.,31.8709650095283));
#19531=CARTESIAN_POINT('',(-1.,1.,32.0051391577542));
#19532=CARTESIAN_POINT('',(-1.,-1.,31.8709650095283));
#19533=CARTESIAN_POINT('Origin',(-1.45,-1.,31.7071784041085));
#19534=CARTESIAN_POINT('',(-1.45,-1.,31.7071784041085));
#19535=CARTESIAN_POINT('',(-1.,-1.,31.8709650095283));
#19536=CARTESIAN_POINT('',(-1.45,1.,31.7071784041085));
#19537=CARTESIAN_POINT('',(-1.,1.,31.8709650095283));
#19538=CARTESIAN_POINT('',(-1.45,-1.,31.7071784041085));
#19539=CARTESIAN_POINT('Origin',(-1.45,-1.,31.540607232456));
#19540=CARTESIAN_POINT('',(-1.45,-1.,31.540607232456));
#19541=CARTESIAN_POINT('',(-1.45,-1.,31.7071784041085));
#19542=CARTESIAN_POINT('',(-1.45,1.,31.540607232456));
#19543=CARTESIAN_POINT('',(-1.45,1.,31.7071784041085));
#19544=CARTESIAN_POINT('',(-1.45,-1.,31.540607232456));
#19545=CARTESIAN_POINT('Origin',(-1.,-1.,31.3768206270362));
#19546=CARTESIAN_POINT('',(-1.,-1.,31.3768206270362));
#19547=CARTESIAN_POINT('',(-1.45,-1.,31.540607232456));
#19548=CARTESIAN_POINT('',(-1.,1.,31.3768206270362));
#19549=CARTESIAN_POINT('',(-1.45,1.,31.540607232456));
#19550=CARTESIAN_POINT('',(-1.,-1.,31.3768206270362));
#19551=CARTESIAN_POINT('Origin',(-1.,-1.,31.2426464788103));
#19552=CARTESIAN_POINT('',(-1.,-1.,31.2426464788103));
#19553=CARTESIAN_POINT('',(-1.,-1.,31.3768206270362));
#19554=CARTESIAN_POINT('',(-1.,1.,31.2426464788103));
#19555=CARTESIAN_POINT('',(-1.,1.,31.3768206270362));
#19556=CARTESIAN_POINT('',(-1.,-1.,31.2426464788103));
#19557=CARTESIAN_POINT('Origin',(-1.45,-1.,31.0788598733905));
#19558=CARTESIAN_POINT('',(-1.45,-1.,31.0788598733905));
#19559=CARTESIAN_POINT('',(-1.,-1.,31.2426464788103));
#19560=CARTESIAN_POINT('',(-1.45,1.,31.0788598733905));
#19561=CARTESIAN_POINT('',(-1.,1.,31.2426464788103));
#19562=CARTESIAN_POINT('',(-1.45,-1.,31.0788598733905));
#19563=CARTESIAN_POINT('Origin',(-1.45,-1.,30.912288701738));
#19564=CARTESIAN_POINT('',(-1.45,-1.,30.912288701738));
#19565=CARTESIAN_POINT('',(-1.45,-1.,31.0788598733905));
#19566=CARTESIAN_POINT('',(-1.45,1.,30.912288701738));
#19567=CARTESIAN_POINT('',(-1.45,1.,31.0788598733905));
#19568=CARTESIAN_POINT('',(-1.45,-1.,30.912288701738));
#19569=CARTESIAN_POINT('Origin',(-1.,-1.,30.7485020963182));
#19570=CARTESIAN_POINT('',(-1.,-1.,30.7485020963182));
#19571=CARTESIAN_POINT('',(-1.45,-1.,30.912288701738));
#19572=CARTESIAN_POINT('',(-1.,1.,30.7485020963182));
#19573=CARTESIAN_POINT('',(-1.45,1.,30.912288701738));
#19574=CARTESIAN_POINT('',(-1.,-1.,30.7485020963182));
#19575=CARTESIAN_POINT('Origin',(-1.,-1.,30.6143279480924));
#19576=CARTESIAN_POINT('',(-1.,-1.,30.6143279480924));
#19577=CARTESIAN_POINT('',(-1.,-1.,30.7485020963182));
#19578=CARTESIAN_POINT('',(-1.,1.,30.6143279480924));
#19579=CARTESIAN_POINT('',(-1.,1.,30.7485020963182));
#19580=CARTESIAN_POINT('',(-1.,-1.,30.6143279480924));
#19581=CARTESIAN_POINT('Origin',(-1.45,-1.,30.4505413426726));
#19582=CARTESIAN_POINT('',(-1.45,-1.,30.4505413426726));
#19583=CARTESIAN_POINT('',(-1.,-1.,30.6143279480924));
#19584=CARTESIAN_POINT('',(-1.45,1.,30.4505413426726));
#19585=CARTESIAN_POINT('',(-1.,1.,30.6143279480924));
#19586=CARTESIAN_POINT('',(-1.45,-1.,30.4505413426726));
#19587=CARTESIAN_POINT('Origin',(-1.45,-1.,30.2839701710201));
#19588=CARTESIAN_POINT('',(-1.45,-1.,30.2839701710201));
#19589=CARTESIAN_POINT('',(-1.45,-1.,30.4505413426726));
#19590=CARTESIAN_POINT('',(-1.45,1.,30.2839701710201));
#19591=CARTESIAN_POINT('',(-1.45,1.,30.4505413426726));
#19592=CARTESIAN_POINT('',(-1.45,-1.,30.2839701710201));
#19593=CARTESIAN_POINT('Origin',(-1.,-1.,30.1201835656003));
#19594=CARTESIAN_POINT('',(-1.,-1.,30.1201835656003));
#19595=CARTESIAN_POINT('',(-1.45,-1.,30.2839701710201));
#19596=CARTESIAN_POINT('',(-1.,1.,30.1201835656003));
#19597=CARTESIAN_POINT('',(-1.45,1.,30.2839701710201));
#19598=CARTESIAN_POINT('',(-1.,-1.,30.1201835656003));
#19599=CARTESIAN_POINT('Origin',(-1.,-1.,29.9860094173744));
#19600=CARTESIAN_POINT('',(-1.,-1.,29.9860094173744));
#19601=CARTESIAN_POINT('',(-1.,-1.,30.1201835656003));
#19602=CARTESIAN_POINT('',(-1.,1.,29.9860094173744));
#19603=CARTESIAN_POINT('',(-1.,1.,30.1201835656003));
#19604=CARTESIAN_POINT('',(-1.,-1.,29.9860094173744));
#19605=CARTESIAN_POINT('Origin',(-1.45,-1.,29.8222228119546));
#19606=CARTESIAN_POINT('',(-1.45,-1.,29.8222228119546));
#19607=CARTESIAN_POINT('',(-1.,-1.,29.9860094173744));
#19608=CARTESIAN_POINT('',(-1.45,1.,29.8222228119546));
#19609=CARTESIAN_POINT('',(-1.,1.,29.9860094173744));
#19610=CARTESIAN_POINT('',(-1.45,-1.,29.8222228119546));
#19611=CARTESIAN_POINT('Origin',(-1.45,-1.,29.6556516403021));
#19612=CARTESIAN_POINT('',(-1.45,-1.,29.6556516403021));
#19613=CARTESIAN_POINT('',(-1.45,-1.,29.8222228119546));
#19614=CARTESIAN_POINT('',(-1.45,1.,29.6556516403021));
#19615=CARTESIAN_POINT('',(-1.45,1.,29.8222228119546));
#19616=CARTESIAN_POINT('',(-1.45,-1.,29.6556516403021));
#19617=CARTESIAN_POINT('Origin',(-1.,-1.,29.4918650348823));
#19618=CARTESIAN_POINT('',(-1.,-1.,29.4918650348823));
#19619=CARTESIAN_POINT('',(-1.45,-1.,29.6556516403021));
#19620=CARTESIAN_POINT('',(-1.,1.,29.4918650348823));
#19621=CARTESIAN_POINT('',(-1.45,1.,29.6556516403021));
#19622=CARTESIAN_POINT('',(-1.,-1.,29.4918650348823));
#19623=CARTESIAN_POINT('Origin',(-1.,-1.,29.3576908866564));
#19624=CARTESIAN_POINT('',(-1.,-1.,29.3576908866564));
#19625=CARTESIAN_POINT('',(-1.,-1.,29.4918650348823));
#19626=CARTESIAN_POINT('',(-1.,1.,29.3576908866564));
#19627=CARTESIAN_POINT('',(-1.,1.,29.4918650348823));
#19628=CARTESIAN_POINT('',(-1.,-1.,29.3576908866564));
#19629=CARTESIAN_POINT('Origin',(-1.45,-1.,29.1939042812366));
#19630=CARTESIAN_POINT('',(-1.45,-1.,29.1939042812366));
#19631=CARTESIAN_POINT('',(-1.,-1.,29.3576908866564));
#19632=CARTESIAN_POINT('',(-1.45,1.,29.1939042812366));
#19633=CARTESIAN_POINT('',(-1.,1.,29.3576908866564));
#19634=CARTESIAN_POINT('',(-1.45,-1.,29.1939042812366));
#19635=CARTESIAN_POINT('Origin',(-1.45,-1.,29.0273331095841));
#19636=CARTESIAN_POINT('',(-1.45,-1.,29.0273331095841));
#19637=CARTESIAN_POINT('',(-1.45,-1.,29.1939042812366));
#19638=CARTESIAN_POINT('',(-1.45,1.,29.0273331095841));
#19639=CARTESIAN_POINT('',(-1.45,1.,29.1939042812366));
#19640=CARTESIAN_POINT('',(-1.45,-1.,29.0273331095841));
#19641=CARTESIAN_POINT('Origin',(-1.,-1.,28.8635465041644));
#19642=CARTESIAN_POINT('',(-1.,-1.,28.8635465041644));
#19643=CARTESIAN_POINT('',(-1.45,-1.,29.0273331095841));
#19644=CARTESIAN_POINT('',(-1.,1.,28.8635465041644));
#19645=CARTESIAN_POINT('',(-1.45,1.,29.0273331095841));
#19646=CARTESIAN_POINT('',(-1.,-1.,28.8635465041644));
#19647=CARTESIAN_POINT('Origin',(-1.,-1.,28.7293723559385));
#19648=CARTESIAN_POINT('',(-1.,-1.,28.7293723559385));
#19649=CARTESIAN_POINT('',(-1.,-1.,28.8635465041644));
#19650=CARTESIAN_POINT('',(-1.,1.,28.7293723559385));
#19651=CARTESIAN_POINT('',(-1.,1.,28.8635465041644));
#19652=CARTESIAN_POINT('',(-1.,-1.,28.7293723559385));
#19653=CARTESIAN_POINT('Origin',(-1.45,-1.,28.5655857505187));
#19654=CARTESIAN_POINT('',(-1.45,-1.,28.5655857505187));
#19655=CARTESIAN_POINT('',(-1.,-1.,28.7293723559385));
#19656=CARTESIAN_POINT('',(-1.45,1.,28.5655857505187));
#19657=CARTESIAN_POINT('',(-1.,1.,28.7293723559385));
#19658=CARTESIAN_POINT('',(-1.45,-1.,28.5655857505187));
#19659=CARTESIAN_POINT('Origin',(-1.45,-1.,28.3990145788662));
#19660=CARTESIAN_POINT('',(-1.45,-1.,28.3990145788662));
#19661=CARTESIAN_POINT('',(-1.45,-1.,28.5655857505187));
#19662=CARTESIAN_POINT('',(-1.45,1.,28.3990145788662));
#19663=CARTESIAN_POINT('',(-1.45,1.,28.5655857505187));
#19664=CARTESIAN_POINT('',(-1.45,-1.,28.3990145788662));
#19665=CARTESIAN_POINT('Origin',(-1.,-1.,28.2352279734464));
#19666=CARTESIAN_POINT('',(-1.,-1.,28.2352279734464));
#19667=CARTESIAN_POINT('',(-1.45,-1.,28.3990145788662));
#19668=CARTESIAN_POINT('',(-1.,1.,28.2352279734464));
#19669=CARTESIAN_POINT('',(-1.45,1.,28.3990145788662));
#19670=CARTESIAN_POINT('',(-1.,-1.,28.2352279734464));
#19671=CARTESIAN_POINT('Origin',(-1.,-1.,28.1010538252205));
#19672=CARTESIAN_POINT('',(-1.,-1.,28.1010538252205));
#19673=CARTESIAN_POINT('',(-1.,-1.,28.2352279734464));
#19674=CARTESIAN_POINT('',(-1.,1.,28.1010538252205));
#19675=CARTESIAN_POINT('',(-1.,1.,28.2352279734464));
#19676=CARTESIAN_POINT('',(-1.,-1.,28.1010538252205));
#19677=CARTESIAN_POINT('Origin',(-1.45,-1.,27.9372672198007));
#19678=CARTESIAN_POINT('',(-1.45,-1.,27.9372672198007));
#19679=CARTESIAN_POINT('',(-1.,-1.,28.1010538252205));
#19680=CARTESIAN_POINT('',(-1.45,1.,27.9372672198007));
#19681=CARTESIAN_POINT('',(-1.,1.,28.1010538252205));
#19682=CARTESIAN_POINT('',(-1.45,-1.,27.9372672198007));
#19683=CARTESIAN_POINT('Origin',(-1.45,-1.,27.7706960481482));
#19684=CARTESIAN_POINT('',(-1.45,-1.,27.7706960481482));
#19685=CARTESIAN_POINT('',(-1.45,-1.,27.9372672198007));
#19686=CARTESIAN_POINT('',(-1.45,1.,27.7706960481482));
#19687=CARTESIAN_POINT('',(-1.45,1.,27.9372672198007));
#19688=CARTESIAN_POINT('',(-1.45,-1.,27.7706960481482));
#19689=CARTESIAN_POINT('Origin',(-1.,-1.,27.6069094427284));
#19690=CARTESIAN_POINT('',(-1.,-1.,27.6069094427284));
#19691=CARTESIAN_POINT('',(-1.45,-1.,27.7706960481482));
#19692=CARTESIAN_POINT('',(-1.,1.,27.6069094427284));
#19693=CARTESIAN_POINT('',(-1.45,1.,27.7706960481482));
#19694=CARTESIAN_POINT('',(-1.,-1.,27.6069094427284));
#19695=CARTESIAN_POINT('Origin',(-1.,-1.,27.4727352945026));
#19696=CARTESIAN_POINT('',(-1.,-1.,27.4727352945026));
#19697=CARTESIAN_POINT('',(-1.,-1.,27.6069094427284));
#19698=CARTESIAN_POINT('',(-1.,1.,27.4727352945026));
#19699=CARTESIAN_POINT('',(-1.,1.,27.6069094427284));
#19700=CARTESIAN_POINT('',(-1.,-1.,27.4727352945026));
#19701=CARTESIAN_POINT('Origin',(-1.45,-1.,27.3089486890828));
#19702=CARTESIAN_POINT('',(-1.45,-1.,27.3089486890828));
#19703=CARTESIAN_POINT('',(-1.,-1.,27.4727352945026));
#19704=CARTESIAN_POINT('',(-1.45,1.,27.3089486890828));
#19705=CARTESIAN_POINT('',(-1.,1.,27.4727352945026));
#19706=CARTESIAN_POINT('',(-1.45,-1.,27.3089486890828));
#19707=CARTESIAN_POINT('Origin',(-1.45,-1.,27.1423775174303));
#19708=CARTESIAN_POINT('',(-1.45,-1.,27.1423775174303));
#19709=CARTESIAN_POINT('',(-1.45,-1.,27.3089486890828));
#19710=CARTESIAN_POINT('',(-1.45,1.,27.1423775174303));
#19711=CARTESIAN_POINT('',(-1.45,1.,27.3089486890828));
#19712=CARTESIAN_POINT('',(-1.45,-1.,27.1423775174303));
#19713=CARTESIAN_POINT('Origin',(-1.,-1.,26.9785909120105));
#19714=CARTESIAN_POINT('',(-1.,-1.,26.9785909120105));
#19715=CARTESIAN_POINT('',(-1.45,-1.,27.1423775174303));
#19716=CARTESIAN_POINT('',(-1.,1.,26.9785909120105));
#19717=CARTESIAN_POINT('',(-1.45,1.,27.1423775174303));
#19718=CARTESIAN_POINT('',(-1.,-1.,26.9785909120105));
#19719=CARTESIAN_POINT('Origin',(-1.,-1.,26.8444167637846));
#19720=CARTESIAN_POINT('',(-1.,-1.,26.8444167637846));
#19721=CARTESIAN_POINT('',(-1.,-1.,26.9785909120105));
#19722=CARTESIAN_POINT('',(-1.,1.,26.8444167637846));
#19723=CARTESIAN_POINT('',(-1.,1.,26.9785909120105));
#19724=CARTESIAN_POINT('',(-1.,-1.,26.8444167637846));
#19725=CARTESIAN_POINT('Origin',(-1.45,-1.,26.6806301583648));
#19726=CARTESIAN_POINT('',(-1.45,-1.,26.6806301583648));
#19727=CARTESIAN_POINT('',(-1.,-1.,26.8444167637846));
#19728=CARTESIAN_POINT('',(-1.45,1.,26.6806301583648));
#19729=CARTESIAN_POINT('',(-1.,1.,26.8444167637846));
#19730=CARTESIAN_POINT('',(-1.45,-1.,26.6806301583648));
#19731=CARTESIAN_POINT('Origin',(-1.45,-1.,26.5140589867123));
#19732=CARTESIAN_POINT('',(-1.45,-1.,26.5140589867123));
#19733=CARTESIAN_POINT('',(-1.45,-1.,26.6806301583648));
#19734=CARTESIAN_POINT('',(-1.45,1.,26.5140589867123));
#19735=CARTESIAN_POINT('',(-1.45,1.,26.6806301583648));
#19736=CARTESIAN_POINT('',(-1.45,-1.,26.5140589867123));
#19737=CARTESIAN_POINT('Origin',(-1.,-1.,26.3502723812925));
#19738=CARTESIAN_POINT('',(-1.,-1.,26.3502723812925));
#19739=CARTESIAN_POINT('',(-1.45,-1.,26.5140589867123));
#19740=CARTESIAN_POINT('',(-1.,1.,26.3502723812925));
#19741=CARTESIAN_POINT('',(-1.45,1.,26.5140589867123));
#19742=CARTESIAN_POINT('',(-1.,-1.,26.3502723812925));
#19743=CARTESIAN_POINT('Origin',(-1.,-1.,26.2160982330666));
#19744=CARTESIAN_POINT('',(-1.,-1.,26.2160982330666));
#19745=CARTESIAN_POINT('',(-1.,-1.,26.3502723812925));
#19746=CARTESIAN_POINT('',(-1.,1.,26.2160982330666));
#19747=CARTESIAN_POINT('',(-1.,1.,26.3502723812925));
#19748=CARTESIAN_POINT('',(-1.,-1.,26.2160982330666));
#19749=CARTESIAN_POINT('Origin',(-1.45,-1.,26.0523116276469));
#19750=CARTESIAN_POINT('',(-1.45,-1.,26.0523116276469));
#19751=CARTESIAN_POINT('',(-1.,-1.,26.2160982330666));
#19752=CARTESIAN_POINT('',(-1.45,1.,26.0523116276469));
#19753=CARTESIAN_POINT('',(-1.,1.,26.2160982330666));
#19754=CARTESIAN_POINT('',(-1.45,-1.,26.0523116276469));
#19755=CARTESIAN_POINT('Origin',(-1.45,-1.,25.8857404559944));
#19756=CARTESIAN_POINT('',(-1.45,-1.,25.8857404559944));
#19757=CARTESIAN_POINT('',(-1.45,-1.,26.0523116276469));
#19758=CARTESIAN_POINT('',(-1.45,1.,25.8857404559944));
#19759=CARTESIAN_POINT('',(-1.45,1.,26.0523116276469));
#19760=CARTESIAN_POINT('',(-1.45,-1.,25.8857404559944));
#19761=CARTESIAN_POINT('Origin',(-1.,-1.,25.7219538505746));
#19762=CARTESIAN_POINT('',(-1.,-1.,25.7219538505746));
#19763=CARTESIAN_POINT('',(-1.45,-1.,25.8857404559944));
#19764=CARTESIAN_POINT('',(-1.,1.,25.7219538505746));
#19765=CARTESIAN_POINT('',(-1.45,1.,25.8857404559944));
#19766=CARTESIAN_POINT('',(-1.,-1.,25.7219538505746));
#19767=CARTESIAN_POINT('Origin',(-1.,-1.,25.5877797023487));
#19768=CARTESIAN_POINT('',(-1.,-1.,25.5877797023487));
#19769=CARTESIAN_POINT('',(-1.,-1.,25.7219538505746));
#19770=CARTESIAN_POINT('',(-1.,1.,25.5877797023487));
#19771=CARTESIAN_POINT('',(-1.,1.,25.7219538505746));
#19772=CARTESIAN_POINT('',(-1.,-1.,25.5877797023487));
#19773=CARTESIAN_POINT('Origin',(-1.45,-1.,25.4239930969289));
#19774=CARTESIAN_POINT('',(-1.45,-1.,25.4239930969289));
#19775=CARTESIAN_POINT('',(-1.,-1.,25.5877797023487));
#19776=CARTESIAN_POINT('',(-1.45,1.,25.4239930969289));
#19777=CARTESIAN_POINT('',(-1.,1.,25.5877797023487));
#19778=CARTESIAN_POINT('',(-1.45,-1.,25.4239930969289));
#19779=CARTESIAN_POINT('Origin',(-1.45,-1.,25.2574219252764));
#19780=CARTESIAN_POINT('',(-1.45,-1.,25.2574219252764));
#19781=CARTESIAN_POINT('',(-1.45,-1.,25.4239930969289));
#19782=CARTESIAN_POINT('',(-1.45,1.,25.2574219252764));
#19783=CARTESIAN_POINT('',(-1.45,1.,25.4239930969289));
#19784=CARTESIAN_POINT('',(-1.45,-1.,25.2574219252764));
#19785=CARTESIAN_POINT('Origin',(-1.,-1.,25.0936353198566));
#19786=CARTESIAN_POINT('',(-1.,-1.,25.0936353198566));
#19787=CARTESIAN_POINT('',(-1.45,-1.,25.2574219252764));
#19788=CARTESIAN_POINT('',(-1.,1.,25.0936353198566));
#19789=CARTESIAN_POINT('',(-1.45,1.,25.2574219252764));
#19790=CARTESIAN_POINT('',(-1.,-1.,25.0936353198566));
#19791=CARTESIAN_POINT('Origin',(-1.,-1.,24.9594611716307));
#19792=CARTESIAN_POINT('',(-1.,-1.,24.9594611716307));
#19793=CARTESIAN_POINT('',(-1.,-1.,25.0936353198566));
#19794=CARTESIAN_POINT('',(-1.,1.,24.9594611716307));
#19795=CARTESIAN_POINT('',(-1.,1.,25.0936353198566));
#19796=CARTESIAN_POINT('',(-1.,-1.,24.9594611716307));
#19797=CARTESIAN_POINT('Origin',(-1.45,-1.,24.7956745662109));
#19798=CARTESIAN_POINT('',(-1.45,-1.,24.7956745662109));
#19799=CARTESIAN_POINT('',(-1.,-1.,24.9594611716307));
#19800=CARTESIAN_POINT('',(-1.45,1.,24.7956745662109));
#19801=CARTESIAN_POINT('',(-1.,1.,24.9594611716307));
#19802=CARTESIAN_POINT('',(-1.45,-1.,24.7956745662109));
#19803=CARTESIAN_POINT('Origin',(-1.45,-1.,24.6291033945584));
#19804=CARTESIAN_POINT('',(-1.45,-1.,24.6291033945584));
#19805=CARTESIAN_POINT('',(-1.45,-1.,24.7956745662109));
#19806=CARTESIAN_POINT('',(-1.45,1.,24.6291033945584));
#19807=CARTESIAN_POINT('',(-1.45,1.,24.7956745662109));
#19808=CARTESIAN_POINT('',(-1.45,-1.,24.6291033945584));
#19809=CARTESIAN_POINT('Origin',(-1.,-1.,24.4653167891386));
#19810=CARTESIAN_POINT('',(-1.,-1.,24.4653167891386));
#19811=CARTESIAN_POINT('',(-1.45,-1.,24.6291033945584));
#19812=CARTESIAN_POINT('',(-1.,1.,24.4653167891386));
#19813=CARTESIAN_POINT('',(-1.45,1.,24.6291033945584));
#19814=CARTESIAN_POINT('',(-1.,-1.,24.4653167891386));
#19815=CARTESIAN_POINT('Origin',(-1.,-1.,24.3311426409128));
#19816=CARTESIAN_POINT('',(-1.,-1.,24.3311426409128));
#19817=CARTESIAN_POINT('',(-1.,-1.,24.4653167891386));
#19818=CARTESIAN_POINT('',(-1.,1.,24.3311426409128));
#19819=CARTESIAN_POINT('',(-1.,1.,24.4653167891386));
#19820=CARTESIAN_POINT('',(-1.,-1.,24.3311426409128));
#19821=CARTESIAN_POINT('Origin',(-1.45,-1.,24.167356035493));
#19822=CARTESIAN_POINT('',(-1.45,-1.,24.167356035493));
#19823=CARTESIAN_POINT('',(-1.,-1.,24.3311426409128));
#19824=CARTESIAN_POINT('',(-1.45,1.,24.167356035493));
#19825=CARTESIAN_POINT('',(-1.,1.,24.3311426409128));
#19826=CARTESIAN_POINT('',(-1.45,-1.,24.167356035493));
#19827=CARTESIAN_POINT('Origin',(-1.45,-1.,24.0007848638405));
#19828=CARTESIAN_POINT('',(-1.45,-1.,24.0007848638405));
#19829=CARTESIAN_POINT('',(-1.45,-1.,24.167356035493));
#19830=CARTESIAN_POINT('',(-1.45,1.,24.0007848638405));
#19831=CARTESIAN_POINT('',(-1.45,1.,24.167356035493));
#19832=CARTESIAN_POINT('',(-1.45,-1.,24.0007848638405));
#19833=CARTESIAN_POINT('Origin',(-1.,-1.,23.8369982584207));
#19834=CARTESIAN_POINT('',(-1.,-1.,23.8369982584207));
#19835=CARTESIAN_POINT('',(-1.45,-1.,24.0007848638405));
#19836=CARTESIAN_POINT('',(-1.,1.,23.8369982584207));
#19837=CARTESIAN_POINT('',(-1.45,1.,24.0007848638405));
#19838=CARTESIAN_POINT('',(-1.,-1.,23.8369982584207));
#19839=CARTESIAN_POINT('Origin',(-1.,-1.,23.7028241101948));
#19840=CARTESIAN_POINT('',(-1.,-1.,23.7028241101948));
#19841=CARTESIAN_POINT('',(-1.,-1.,23.8369982584207));
#19842=CARTESIAN_POINT('',(-1.,1.,23.7028241101948));
#19843=CARTESIAN_POINT('',(-1.,1.,23.8369982584207));
#19844=CARTESIAN_POINT('',(-1.,-1.,23.7028241101948));
#19845=CARTESIAN_POINT('Origin',(-1.45,-1.,23.539037504775));
#19846=CARTESIAN_POINT('',(-1.45,-1.,23.539037504775));
#19847=CARTESIAN_POINT('',(-1.,-1.,23.7028241101948));
#19848=CARTESIAN_POINT('',(-1.45,1.,23.539037504775));
#19849=CARTESIAN_POINT('',(-1.,1.,23.7028241101948));
#19850=CARTESIAN_POINT('',(-1.45,-1.,23.539037504775));
#19851=CARTESIAN_POINT('Origin',(-1.45,-1.,23.3724663331225));
#19852=CARTESIAN_POINT('',(-1.45,-1.,23.3724663331225));
#19853=CARTESIAN_POINT('',(-1.45,-1.,23.539037504775));
#19854=CARTESIAN_POINT('',(-1.45,1.,23.3724663331225));
#19855=CARTESIAN_POINT('',(-1.45,1.,23.539037504775));
#19856=CARTESIAN_POINT('',(-1.45,-1.,23.3724663331225));
#19857=CARTESIAN_POINT('Origin',(-1.,-1.,23.2086797277027));
#19858=CARTESIAN_POINT('',(-1.,-1.,23.2086797277027));
#19859=CARTESIAN_POINT('',(-1.45,-1.,23.3724663331225));
#19860=CARTESIAN_POINT('',(-1.,1.,23.2086797277027));
#19861=CARTESIAN_POINT('',(-1.45,1.,23.3724663331225));
#19862=CARTESIAN_POINT('',(-1.,-1.,23.2086797277027));
#19863=CARTESIAN_POINT('Origin',(-1.,-1.,23.0745055794769));
#19864=CARTESIAN_POINT('',(-1.,-1.,23.0745055794769));
#19865=CARTESIAN_POINT('',(-1.,-1.,23.2086797277027));
#19866=CARTESIAN_POINT('',(-1.,1.,23.0745055794769));
#19867=CARTESIAN_POINT('',(-1.,1.,23.2086797277027));
#19868=CARTESIAN_POINT('',(-1.,-1.,23.0745055794769));
#19869=CARTESIAN_POINT('Origin',(-1.45,-1.,22.9107189740571));
#19870=CARTESIAN_POINT('',(-1.45,-1.,22.9107189740571));
#19871=CARTESIAN_POINT('',(-1.,-1.,23.0745055794769));
#19872=CARTESIAN_POINT('',(-1.45,1.,22.9107189740571));
#19873=CARTESIAN_POINT('',(-1.,1.,23.0745055794769));
#19874=CARTESIAN_POINT('',(-1.45,-1.,22.9107189740571));
#19875=CARTESIAN_POINT('Origin',(-1.45,-1.,22.7441478024046));
#19876=CARTESIAN_POINT('',(-1.45,-1.,22.7441478024046));
#19877=CARTESIAN_POINT('',(-1.45,-1.,22.9107189740571));
#19878=CARTESIAN_POINT('',(-1.45,1.,22.7441478024046));
#19879=CARTESIAN_POINT('',(-1.45,1.,22.9107189740571));
#19880=CARTESIAN_POINT('',(-1.45,-1.,22.7441478024046));
#19881=CARTESIAN_POINT('Origin',(-1.,-1.,22.5803611969848));
#19882=CARTESIAN_POINT('',(-1.,-1.,22.5803611969848));
#19883=CARTESIAN_POINT('',(-1.45,-1.,22.7441478024046));
#19884=CARTESIAN_POINT('',(-1.,1.,22.5803611969848));
#19885=CARTESIAN_POINT('',(-1.45,1.,22.7441478024046));
#19886=CARTESIAN_POINT('',(-1.,-1.,22.5803611969848));
#19887=CARTESIAN_POINT('Origin',(-1.,-1.,22.4461870487589));
#19888=CARTESIAN_POINT('',(-1.,-1.,22.4461870487589));
#19889=CARTESIAN_POINT('',(-1.,-1.,22.5803611969848));
#19890=CARTESIAN_POINT('',(-1.,1.,22.4461870487589));
#19891=CARTESIAN_POINT('',(-1.,1.,22.5803611969848));
#19892=CARTESIAN_POINT('',(-1.,-1.,22.4461870487589));
#19893=CARTESIAN_POINT('Origin',(-1.45,-1.,22.2824004433391));
#19894=CARTESIAN_POINT('',(-1.45,-1.,22.2824004433391));
#19895=CARTESIAN_POINT('',(-1.,-1.,22.4461870487589));
#19896=CARTESIAN_POINT('',(-1.45,1.,22.2824004433391));
#19897=CARTESIAN_POINT('',(-1.,1.,22.4461870487589));
#19898=CARTESIAN_POINT('',(-1.45,-1.,22.2824004433391));
#19899=CARTESIAN_POINT('Origin',(-1.45,-1.,22.1158292716866));
#19900=CARTESIAN_POINT('',(-1.45,-1.,22.1158292716866));
#19901=CARTESIAN_POINT('',(-1.45,-1.,22.2824004433391));
#19902=CARTESIAN_POINT('',(-1.45,1.,22.1158292716866));
#19903=CARTESIAN_POINT('',(-1.45,1.,22.2824004433391));
#19904=CARTESIAN_POINT('',(-1.45,-1.,22.1158292716866));
#19905=CARTESIAN_POINT('Origin',(-1.,-1.,21.9520426662668));
#19906=CARTESIAN_POINT('',(-1.,-1.,21.9520426662668));
#19907=CARTESIAN_POINT('',(-1.45,-1.,22.1158292716866));
#19908=CARTESIAN_POINT('',(-1.,1.,21.9520426662668));
#19909=CARTESIAN_POINT('',(-1.45,1.,22.1158292716866));
#19910=CARTESIAN_POINT('',(-1.,-1.,21.9520426662668));
#19911=CARTESIAN_POINT('Origin',(-1.,-1.,21.8178685180409));
#19912=CARTESIAN_POINT('',(-1.,-1.,21.8178685180409));
#19913=CARTESIAN_POINT('',(-1.,-1.,21.9520426662668));
#19914=CARTESIAN_POINT('',(-1.,1.,21.8178685180409));
#19915=CARTESIAN_POINT('',(-1.,1.,21.9520426662668));
#19916=CARTESIAN_POINT('',(-1.,-1.,21.8178685180409));
#19917=CARTESIAN_POINT('Origin',(-1.45,-1.,21.6540819126211));
#19918=CARTESIAN_POINT('',(-1.45,-1.,21.6540819126211));
#19919=CARTESIAN_POINT('',(-1.,-1.,21.8178685180409));
#19920=CARTESIAN_POINT('',(-1.45,1.,21.6540819126211));
#19921=CARTESIAN_POINT('',(-1.,1.,21.8178685180409));
#19922=CARTESIAN_POINT('',(-1.45,-1.,21.6540819126211));
#19923=CARTESIAN_POINT('Origin',(-1.45,-1.,21.4875107409686));
#19924=CARTESIAN_POINT('',(-1.45,-1.,21.4875107409686));
#19925=CARTESIAN_POINT('',(-1.45,-1.,21.6540819126211));
#19926=CARTESIAN_POINT('',(-1.45,1.,21.4875107409686));
#19927=CARTESIAN_POINT('',(-1.45,1.,21.6540819126211));
#19928=CARTESIAN_POINT('',(-1.45,-1.,21.4875107409686));
#19929=CARTESIAN_POINT('Origin',(-1.,-1.,21.3237241355489));
#19930=CARTESIAN_POINT('',(-1.,-1.,21.3237241355489));
#19931=CARTESIAN_POINT('',(-1.45,-1.,21.4875107409686));
#19932=CARTESIAN_POINT('',(-1.,1.,21.3237241355489));
#19933=CARTESIAN_POINT('',(-1.45,1.,21.4875107409686));
#19934=CARTESIAN_POINT('',(-1.,-1.,21.3237241355489));
#19935=CARTESIAN_POINT('Origin',(-1.,-1.,21.189549987323));
#19936=CARTESIAN_POINT('',(-1.,-1.,21.189549987323));
#19937=CARTESIAN_POINT('',(-1.,-1.,21.3237241355489));
#19938=CARTESIAN_POINT('',(-1.,1.,21.189549987323));
#19939=CARTESIAN_POINT('',(-1.,1.,21.3237241355489));
#19940=CARTESIAN_POINT('',(-1.,-1.,21.189549987323));
#19941=CARTESIAN_POINT('Origin',(-1.45,-1.,21.0257633819032));
#19942=CARTESIAN_POINT('',(-1.45,-1.,21.0257633819032));
#19943=CARTESIAN_POINT('',(-1.,-1.,21.189549987323));
#19944=CARTESIAN_POINT('',(-1.45,1.,21.0257633819032));
#19945=CARTESIAN_POINT('',(-1.,1.,21.189549987323));
#19946=CARTESIAN_POINT('',(-1.45,-1.,21.0257633819032));
#19947=CARTESIAN_POINT('Origin',(-1.45,-1.,20.8591922102507));
#19948=CARTESIAN_POINT('',(-1.45,-1.,20.8591922102507));
#19949=CARTESIAN_POINT('',(-1.45,-1.,21.0257633819032));
#19950=CARTESIAN_POINT('',(-1.45,1.,20.8591922102507));
#19951=CARTESIAN_POINT('',(-1.45,1.,21.0257633819032));
#19952=CARTESIAN_POINT('',(-1.45,-1.,20.8591922102507));
#19953=CARTESIAN_POINT('Origin',(-1.,-1.,20.6954056048309));
#19954=CARTESIAN_POINT('',(-1.,-1.,20.6954056048309));
#19955=CARTESIAN_POINT('',(-1.45,-1.,20.8591922102507));
#19956=CARTESIAN_POINT('',(-1.,1.,20.6954056048309));
#19957=CARTESIAN_POINT('',(-1.45,1.,20.8591922102507));
#19958=CARTESIAN_POINT('',(-1.,-1.,20.6954056048309));
#19959=CARTESIAN_POINT('Origin',(-1.,-1.,20.561231456605));
#19960=CARTESIAN_POINT('',(-1.,-1.,20.561231456605));
#19961=CARTESIAN_POINT('',(-1.,-1.,20.6954056048309));
#19962=CARTESIAN_POINT('',(-1.,1.,20.561231456605));
#19963=CARTESIAN_POINT('',(-1.,1.,20.6954056048309));
#19964=CARTESIAN_POINT('',(-1.,-1.,20.561231456605));
#19965=CARTESIAN_POINT('Origin',(-1.45,-1.,20.3974448511852));
#19966=CARTESIAN_POINT('',(-1.45,-1.,20.3974448511852));
#19967=CARTESIAN_POINT('',(-1.,-1.,20.561231456605));
#19968=CARTESIAN_POINT('',(-1.45,1.,20.3974448511852));
#19969=CARTESIAN_POINT('',(-1.,1.,20.561231456605));
#19970=CARTESIAN_POINT('',(-1.45,-1.,20.3974448511852));
#19971=CARTESIAN_POINT('Origin',(-1.45,-1.,20.2308736795327));
#19972=CARTESIAN_POINT('',(-1.45,-1.,20.2308736795327));
#19973=CARTESIAN_POINT('',(-1.45,-1.,20.3974448511852));
#19974=CARTESIAN_POINT('',(-1.45,1.,20.2308736795327));
#19975=CARTESIAN_POINT('',(-1.45,1.,20.3974448511852));
#19976=CARTESIAN_POINT('',(-1.45,-1.,20.2308736795327));
#19977=CARTESIAN_POINT('Origin',(-1.,-1.,20.0670870741129));
#19978=CARTESIAN_POINT('',(-1.,-1.,20.0670870741129));
#19979=CARTESIAN_POINT('',(-1.45,-1.,20.2308736795327));
#19980=CARTESIAN_POINT('',(-1.,1.,20.0670870741129));
#19981=CARTESIAN_POINT('',(-1.45,1.,20.2308736795327));
#19982=CARTESIAN_POINT('',(-1.,-1.,20.0670870741129));
#19983=CARTESIAN_POINT('Origin',(-1.,-1.,19.9329129258871));
#19984=CARTESIAN_POINT('',(-1.,-1.,19.9329129258871));
#19985=CARTESIAN_POINT('',(-1.,-1.,20.0670870741129));
#19986=CARTESIAN_POINT('',(-1.,1.,19.9329129258871));
#19987=CARTESIAN_POINT('',(-1.,1.,20.0670870741129));
#19988=CARTESIAN_POINT('',(-1.,-1.,19.9329129258871));
#19989=CARTESIAN_POINT('Origin',(-1.45,-1.,19.7691263204673));
#19990=CARTESIAN_POINT('',(-1.45,-1.,19.7691263204673));
#19991=CARTESIAN_POINT('',(-1.,-1.,19.9329129258871));
#19992=CARTESIAN_POINT('',(-1.45,1.,19.7691263204673));
#19993=CARTESIAN_POINT('',(-1.,1.,19.9329129258871));
#19994=CARTESIAN_POINT('',(-1.45,-1.,19.7691263204673));
#19995=CARTESIAN_POINT('Origin',(-1.45,-1.,19.6025551488148));
#19996=CARTESIAN_POINT('',(-1.45,-1.,19.6025551488148));
#19997=CARTESIAN_POINT('',(-1.45,-1.,19.7691263204673));
#19998=CARTESIAN_POINT('',(-1.45,1.,19.6025551488148));
#19999=CARTESIAN_POINT('',(-1.45,1.,19.7691263204673));
#20000=CARTESIAN_POINT('',(-1.45,-1.,19.6025551488148));
#20001=CARTESIAN_POINT('Origin',(-1.,-1.,19.438768543395));
#20002=CARTESIAN_POINT('',(-1.,-1.,19.438768543395));
#20003=CARTESIAN_POINT('',(-1.45,-1.,19.6025551488148));
#20004=CARTESIAN_POINT('',(-1.,1.,19.438768543395));
#20005=CARTESIAN_POINT('',(-1.45,1.,19.6025551488148));
#20006=CARTESIAN_POINT('',(-1.,-1.,19.438768543395));
#20007=CARTESIAN_POINT('Origin',(-1.,-1.,19.3045943951691));
#20008=CARTESIAN_POINT('',(-1.,-1.,19.3045943951691));
#20009=CARTESIAN_POINT('',(-1.,-1.,19.438768543395));
#20010=CARTESIAN_POINT('',(-1.,1.,19.3045943951691));
#20011=CARTESIAN_POINT('',(-1.,1.,19.438768543395));
#20012=CARTESIAN_POINT('',(-1.,-1.,19.3045943951691));
#20013=CARTESIAN_POINT('Origin',(-1.45,-1.,19.1408077897493));
#20014=CARTESIAN_POINT('',(-1.45,-1.,19.1408077897493));
#20015=CARTESIAN_POINT('',(-1.,-1.,19.3045943951691));
#20016=CARTESIAN_POINT('',(-1.45,1.,19.1408077897493));
#20017=CARTESIAN_POINT('',(-1.,1.,19.3045943951691));
#20018=CARTESIAN_POINT('',(-1.45,-1.,19.1408077897493));
#20019=CARTESIAN_POINT('Origin',(-1.45,-1.,18.9742366180968));
#20020=CARTESIAN_POINT('',(-1.45,-1.,18.9742366180968));
#20021=CARTESIAN_POINT('',(-1.45,-1.,19.1408077897493));
#20022=CARTESIAN_POINT('',(-1.45,1.,18.9742366180968));
#20023=CARTESIAN_POINT('',(-1.45,1.,19.1408077897493));
#20024=CARTESIAN_POINT('',(-1.45,-1.,18.9742366180968));
#20025=CARTESIAN_POINT('Origin',(-1.,-1.,18.810450012677));
#20026=CARTESIAN_POINT('',(-1.,-1.,18.810450012677));
#20027=CARTESIAN_POINT('',(-1.45,-1.,18.9742366180968));
#20028=CARTESIAN_POINT('',(-1.,1.,18.810450012677));
#20029=CARTESIAN_POINT('',(-1.45,1.,18.9742366180968));
#20030=CARTESIAN_POINT('',(-1.,-1.,18.810450012677));
#20031=CARTESIAN_POINT('Origin',(-1.,-1.,18.6762758644511));
#20032=CARTESIAN_POINT('',(-1.,-1.,18.6762758644511));
#20033=CARTESIAN_POINT('',(-1.,-1.,18.810450012677));
#20034=CARTESIAN_POINT('',(-1.,1.,18.6762758644511));
#20035=CARTESIAN_POINT('',(-1.,1.,18.810450012677));
#20036=CARTESIAN_POINT('',(-1.,-1.,18.6762758644511));
#20037=CARTESIAN_POINT('Origin',(-1.45,-1.,18.5124892590314));
#20038=CARTESIAN_POINT('',(-1.45,-1.,18.5124892590314));
#20039=CARTESIAN_POINT('',(-1.,-1.,18.6762758644511));
#20040=CARTESIAN_POINT('',(-1.45,1.,18.5124892590314));
#20041=CARTESIAN_POINT('',(-1.,1.,18.6762758644511));
#20042=CARTESIAN_POINT('',(-1.45,-1.,18.5124892590314));
#20043=CARTESIAN_POINT('Origin',(-1.45,-1.,18.3459180873789));
#20044=CARTESIAN_POINT('',(-1.45,-1.,18.3459180873789));
#20045=CARTESIAN_POINT('',(-1.45,-1.,18.5124892590314));
#20046=CARTESIAN_POINT('',(-1.45,1.,18.3459180873789));
#20047=CARTESIAN_POINT('',(-1.45,1.,18.5124892590314));
#20048=CARTESIAN_POINT('',(-1.45,-1.,18.3459180873789));
#20049=CARTESIAN_POINT('Origin',(-1.,-1.,18.1821314819591));
#20050=CARTESIAN_POINT('',(-1.,-1.,18.1821314819591));
#20051=CARTESIAN_POINT('',(-1.45,-1.,18.3459180873789));
#20052=CARTESIAN_POINT('',(-1.,1.,18.1821314819591));
#20053=CARTESIAN_POINT('',(-1.45,1.,18.3459180873789));
#20054=CARTESIAN_POINT('',(-1.,-1.,18.1821314819591));
#20055=CARTESIAN_POINT('Origin',(-1.,-1.,18.0479573337332));
#20056=CARTESIAN_POINT('',(-1.,-1.,18.0479573337332));
#20057=CARTESIAN_POINT('',(-1.,-1.,18.1821314819591));
#20058=CARTESIAN_POINT('',(-1.,1.,18.0479573337332));
#20059=CARTESIAN_POINT('',(-1.,1.,18.1821314819591));
#20060=CARTESIAN_POINT('',(-1.,-1.,18.0479573337332));
#20061=CARTESIAN_POINT('Origin',(-1.45,-1.,17.8841707283134));
#20062=CARTESIAN_POINT('',(-1.45,-1.,17.8841707283134));
#20063=CARTESIAN_POINT('',(-1.,-1.,18.0479573337332));
#20064=CARTESIAN_POINT('',(-1.45,1.,17.8841707283134));
#20065=CARTESIAN_POINT('',(-1.,1.,18.0479573337332));
#20066=CARTESIAN_POINT('',(-1.45,-1.,17.8841707283134));
#20067=CARTESIAN_POINT('Origin',(-1.45,-1.,17.7175995566609));
#20068=CARTESIAN_POINT('',(-1.45,-1.,17.7175995566609));
#20069=CARTESIAN_POINT('',(-1.45,-1.,17.8841707283134));
#20070=CARTESIAN_POINT('',(-1.45,1.,17.7175995566609));
#20071=CARTESIAN_POINT('',(-1.45,1.,17.8841707283134));
#20072=CARTESIAN_POINT('',(-1.45,-1.,17.7175995566609));
#20073=CARTESIAN_POINT('Origin',(-1.,-1.,17.5538129512411));
#20074=CARTESIAN_POINT('',(-1.,-1.,17.5538129512411));
#20075=CARTESIAN_POINT('',(-1.45,-1.,17.7175995566609));
#20076=CARTESIAN_POINT('',(-1.,1.,17.5538129512411));
#20077=CARTESIAN_POINT('',(-1.45,1.,17.7175995566609));
#20078=CARTESIAN_POINT('',(-1.,-1.,17.5538129512411));
#20079=CARTESIAN_POINT('Origin',(-1.,-1.,17.4196388030152));
#20080=CARTESIAN_POINT('',(-1.,-1.,17.4196388030152));
#20081=CARTESIAN_POINT('',(-1.,-1.,17.5538129512411));
#20082=CARTESIAN_POINT('',(-1.,1.,17.4196388030152));
#20083=CARTESIAN_POINT('',(-1.,1.,17.5538129512411));
#20084=CARTESIAN_POINT('',(-1.,-1.,17.4196388030152));
#20085=CARTESIAN_POINT('Origin',(-1.45,-1.,17.2558521975954));
#20086=CARTESIAN_POINT('',(-1.45,-1.,17.2558521975954));
#20087=CARTESIAN_POINT('',(-1.,-1.,17.4196388030152));
#20088=CARTESIAN_POINT('',(-1.45,1.,17.2558521975954));
#20089=CARTESIAN_POINT('',(-1.,1.,17.4196388030152));
#20090=CARTESIAN_POINT('',(-1.45,-1.,17.2558521975954));
#20091=CARTESIAN_POINT('Origin',(-1.45,-1.,17.0892810259429));
#20092=CARTESIAN_POINT('',(-1.45,-1.,17.0892810259429));
#20093=CARTESIAN_POINT('',(-1.45,-1.,17.2558521975954));
#20094=CARTESIAN_POINT('',(-1.45,1.,17.0892810259429));
#20095=CARTESIAN_POINT('',(-1.45,1.,17.2558521975954));
#20096=CARTESIAN_POINT('',(-1.45,-1.,17.0892810259429));
#20097=CARTESIAN_POINT('Origin',(-1.,-1.,16.9254944205231));
#20098=CARTESIAN_POINT('',(-1.,-1.,16.9254944205231));
#20099=CARTESIAN_POINT('',(-1.45,-1.,17.0892810259429));
#20100=CARTESIAN_POINT('',(-1.,1.,16.9254944205231));
#20101=CARTESIAN_POINT('',(-1.45,1.,17.0892810259429));
#20102=CARTESIAN_POINT('',(-1.,-1.,16.9254944205231));
#20103=CARTESIAN_POINT('Origin',(-1.,-1.,16.7913202722973));
#20104=CARTESIAN_POINT('',(-1.,-1.,16.7913202722973));
#20105=CARTESIAN_POINT('',(-1.,-1.,16.9254944205231));
#20106=CARTESIAN_POINT('',(-1.,1.,16.7913202722973));
#20107=CARTESIAN_POINT('',(-1.,1.,16.9254944205231));
#20108=CARTESIAN_POINT('',(-1.,-1.,16.7913202722973));
#20109=CARTESIAN_POINT('Origin',(-1.45,-1.,16.6275336668775));
#20110=CARTESIAN_POINT('',(-1.45,-1.,16.6275336668775));
#20111=CARTESIAN_POINT('',(-1.,-1.,16.7913202722973));
#20112=CARTESIAN_POINT('',(-1.45,1.,16.6275336668775));
#20113=CARTESIAN_POINT('',(-1.,1.,16.7913202722973));
#20114=CARTESIAN_POINT('',(-1.45,-1.,16.6275336668775));
#20115=CARTESIAN_POINT('Origin',(-1.45,-1.,16.460962495225));
#20116=CARTESIAN_POINT('',(-1.45,-1.,16.460962495225));
#20117=CARTESIAN_POINT('',(-1.45,-1.,16.6275336668775));
#20118=CARTESIAN_POINT('',(-1.45,1.,16.460962495225));
#20119=CARTESIAN_POINT('',(-1.45,1.,16.6275336668775));
#20120=CARTESIAN_POINT('',(-1.45,-1.,16.460962495225));
#20121=CARTESIAN_POINT('Origin',(-1.,-1.,16.2971758898052));
#20122=CARTESIAN_POINT('',(-1.,-1.,16.2971758898052));
#20123=CARTESIAN_POINT('',(-1.45,-1.,16.460962495225));
#20124=CARTESIAN_POINT('',(-1.,1.,16.2971758898052));
#20125=CARTESIAN_POINT('',(-1.45,1.,16.460962495225));
#20126=CARTESIAN_POINT('',(-1.,-1.,16.2971758898052));
#20127=CARTESIAN_POINT('Origin',(-1.,-1.,16.1630017415793));
#20128=CARTESIAN_POINT('',(-1.,-1.,16.1630017415793));
#20129=CARTESIAN_POINT('',(-1.,-1.,16.2971758898052));
#20130=CARTESIAN_POINT('',(-1.,1.,16.1630017415793));
#20131=CARTESIAN_POINT('',(-1.,1.,16.2971758898052));
#20132=CARTESIAN_POINT('',(-1.,-1.,16.1630017415793));
#20133=CARTESIAN_POINT('Origin',(-1.45,-1.,15.9992151361595));
#20134=CARTESIAN_POINT('',(-1.45,-1.,15.9992151361595));
#20135=CARTESIAN_POINT('',(-1.,-1.,16.1630017415793));
#20136=CARTESIAN_POINT('',(-1.45,1.,15.9992151361595));
#20137=CARTESIAN_POINT('',(-1.,1.,16.1630017415793));
#20138=CARTESIAN_POINT('',(-1.45,-1.,15.9992151361595));
#20139=CARTESIAN_POINT('Origin',(-1.45,-1.,15.832643964507));
#20140=CARTESIAN_POINT('',(-1.45,-1.,15.832643964507));
#20141=CARTESIAN_POINT('',(-1.45,-1.,15.9992151361595));
#20142=CARTESIAN_POINT('',(-1.45,1.,15.832643964507));
#20143=CARTESIAN_POINT('',(-1.45,1.,15.9992151361595));
#20144=CARTESIAN_POINT('',(-1.45,-1.,15.832643964507));
#20145=CARTESIAN_POINT('Origin',(-1.,-1.,15.6688573590872));
#20146=CARTESIAN_POINT('',(-1.,-1.,15.6688573590872));
#20147=CARTESIAN_POINT('',(-1.45,-1.,15.832643964507));
#20148=CARTESIAN_POINT('',(-1.,1.,15.6688573590872));
#20149=CARTESIAN_POINT('',(-1.45,1.,15.832643964507));
#20150=CARTESIAN_POINT('',(-1.,-1.,15.6688573590872));
#20151=CARTESIAN_POINT('Origin',(-1.,-1.,15.5346832108613));
#20152=CARTESIAN_POINT('',(-1.,-1.,15.5346832108613));
#20153=CARTESIAN_POINT('',(-1.,-1.,15.6688573590872));
#20154=CARTESIAN_POINT('',(-1.,1.,15.5346832108613));
#20155=CARTESIAN_POINT('',(-1.,1.,15.6688573590872));
#20156=CARTESIAN_POINT('',(-1.,-1.,15.5346832108613));
#20157=CARTESIAN_POINT('Origin',(-1.45,-1.,15.3708966054416));
#20158=CARTESIAN_POINT('',(-1.45,-1.,15.3708966054416));
#20159=CARTESIAN_POINT('',(-1.,-1.,15.5346832108613));
#20160=CARTESIAN_POINT('',(-1.45,1.,15.3708966054416));
#20161=CARTESIAN_POINT('',(-1.,1.,15.5346832108613));
#20162=CARTESIAN_POINT('',(-1.45,-1.,15.3708966054416));
#20163=CARTESIAN_POINT('Origin',(-1.45,-1.,15.2043254337891));
#20164=CARTESIAN_POINT('',(-1.45,-1.,15.2043254337891));
#20165=CARTESIAN_POINT('',(-1.45,-1.,15.3708966054416));
#20166=CARTESIAN_POINT('',(-1.45,1.,15.2043254337891));
#20167=CARTESIAN_POINT('',(-1.45,1.,15.3708966054416));
#20168=CARTESIAN_POINT('',(-1.45,-1.,15.2043254337891));
#20169=CARTESIAN_POINT('Origin',(-1.,-1.,15.0405388283693));
#20170=CARTESIAN_POINT('',(-1.,-1.,15.0405388283693));
#20171=CARTESIAN_POINT('',(-1.45,-1.,15.2043254337891));
#20172=CARTESIAN_POINT('',(-1.,1.,15.0405388283693));
#20173=CARTESIAN_POINT('',(-1.45,1.,15.2043254337891));
#20174=CARTESIAN_POINT('',(-1.,-1.,15.0405388283693));
#20175=CARTESIAN_POINT('Origin',(-1.,-1.,14.9063646801434));
#20176=CARTESIAN_POINT('',(-1.,-1.,14.9063646801434));
#20177=CARTESIAN_POINT('',(-1.,-1.,15.0405388283693));
#20178=CARTESIAN_POINT('',(-1.,1.,14.9063646801434));
#20179=CARTESIAN_POINT('',(-1.,1.,15.0405388283693));
#20180=CARTESIAN_POINT('',(-1.,-1.,14.9063646801434));
#20181=CARTESIAN_POINT('Origin',(-1.45,-1.,14.7425780747236));
#20182=CARTESIAN_POINT('',(-1.45,-1.,14.7425780747236));
#20183=CARTESIAN_POINT('',(-1.,-1.,14.9063646801434));
#20184=CARTESIAN_POINT('',(-1.45,1.,14.7425780747236));
#20185=CARTESIAN_POINT('',(-1.,1.,14.9063646801434));
#20186=CARTESIAN_POINT('',(-1.45,-1.,14.7425780747236));
#20187=CARTESIAN_POINT('Origin',(-1.45,-1.,14.5760069030711));
#20188=CARTESIAN_POINT('',(-1.45,-1.,14.5760069030711));
#20189=CARTESIAN_POINT('',(-1.45,-1.,14.7425780747236));
#20190=CARTESIAN_POINT('',(-1.45,1.,14.5760069030711));
#20191=CARTESIAN_POINT('',(-1.45,1.,14.7425780747236));
#20192=CARTESIAN_POINT('',(-1.45,-1.,14.5760069030711));
#20193=CARTESIAN_POINT('Origin',(-1.,-1.,14.4122202976513));
#20194=CARTESIAN_POINT('',(-1.,-1.,14.4122202976513));
#20195=CARTESIAN_POINT('',(-1.45,-1.,14.5760069030711));
#20196=CARTESIAN_POINT('',(-1.,1.,14.4122202976513));
#20197=CARTESIAN_POINT('',(-1.45,1.,14.5760069030711));
#20198=CARTESIAN_POINT('',(-1.,-1.,14.4122202976513));
#20199=CARTESIAN_POINT('Origin',(-1.,-1.,14.2780461494254));
#20200=CARTESIAN_POINT('',(-1.,-1.,14.2780461494254));
#20201=CARTESIAN_POINT('',(-1.,-1.,14.4122202976513));
#20202=CARTESIAN_POINT('',(-1.,1.,14.2780461494254));
#20203=CARTESIAN_POINT('',(-1.,1.,14.4122202976513));
#20204=CARTESIAN_POINT('',(-1.,-1.,14.2780461494254));
#20205=CARTESIAN_POINT('Origin',(-1.45,-1.,14.1142595440056));
#20206=CARTESIAN_POINT('',(-1.45,-1.,14.1142595440056));
#20207=CARTESIAN_POINT('',(-1.,-1.,14.2780461494254));
#20208=CARTESIAN_POINT('',(-1.45,1.,14.1142595440056));
#20209=CARTESIAN_POINT('',(-1.,1.,14.2780461494254));
#20210=CARTESIAN_POINT('',(-1.45,-1.,14.1142595440056));
#20211=CARTESIAN_POINT('Origin',(-1.45,-1.,13.9476883723531));
#20212=CARTESIAN_POINT('',(-1.45,-1.,13.9476883723531));
#20213=CARTESIAN_POINT('',(-1.45,-1.,14.1142595440056));
#20214=CARTESIAN_POINT('',(-1.45,1.,13.9476883723531));
#20215=CARTESIAN_POINT('',(-1.45,1.,14.1142595440056));
#20216=CARTESIAN_POINT('',(-1.45,-1.,13.9476883723531));
#20217=CARTESIAN_POINT('Origin',(-1.,-1.,13.7839017669334));
#20218=CARTESIAN_POINT('',(-1.,-1.,13.7839017669334));
#20219=CARTESIAN_POINT('',(-1.45,-1.,13.9476883723531));
#20220=CARTESIAN_POINT('',(-1.,1.,13.7839017669334));
#20221=CARTESIAN_POINT('',(-1.45,1.,13.9476883723531));
#20222=CARTESIAN_POINT('',(-1.,-1.,13.7839017669334));
#20223=CARTESIAN_POINT('Origin',(-1.,-1.,13.6497276187075));
#20224=CARTESIAN_POINT('',(-1.,-1.,13.6497276187075));
#20225=CARTESIAN_POINT('',(-1.,-1.,13.7839017669334));
#20226=CARTESIAN_POINT('',(-1.,1.,13.6497276187075));
#20227=CARTESIAN_POINT('',(-1.,1.,13.7839017669334));
#20228=CARTESIAN_POINT('',(-1.,-1.,13.6497276187075));
#20229=CARTESIAN_POINT('Origin',(-1.45,-1.,13.4859410132877));
#20230=CARTESIAN_POINT('',(-1.45,-1.,13.4859410132877));
#20231=CARTESIAN_POINT('',(-1.,-1.,13.6497276187075));
#20232=CARTESIAN_POINT('',(-1.45,1.,13.4859410132877));
#20233=CARTESIAN_POINT('',(-1.,1.,13.6497276187075));
#20234=CARTESIAN_POINT('',(-1.45,-1.,13.4859410132877));
#20235=CARTESIAN_POINT('Origin',(-1.45,-1.,13.3193698416352));
#20236=CARTESIAN_POINT('',(-1.45,-1.,13.3193698416352));
#20237=CARTESIAN_POINT('',(-1.45,-1.,13.4859410132877));
#20238=CARTESIAN_POINT('',(-1.45,1.,13.3193698416352));
#20239=CARTESIAN_POINT('',(-1.45,1.,13.4859410132877));
#20240=CARTESIAN_POINT('',(-1.45,-1.,13.3193698416352));
#20241=CARTESIAN_POINT('Origin',(-1.,-1.,13.1555832362154));
#20242=CARTESIAN_POINT('',(-1.,-1.,13.1555832362154));
#20243=CARTESIAN_POINT('',(-1.45,-1.,13.3193698416352));
#20244=CARTESIAN_POINT('',(-1.,1.,13.1555832362154));
#20245=CARTESIAN_POINT('',(-1.45,1.,13.3193698416352));
#20246=CARTESIAN_POINT('',(-1.,-1.,13.1555832362154));
#20247=CARTESIAN_POINT('Origin',(-1.,-1.,13.0214090879895));
#20248=CARTESIAN_POINT('',(-1.,-1.,13.0214090879895));
#20249=CARTESIAN_POINT('',(-1.,-1.,13.1555832362154));
#20250=CARTESIAN_POINT('',(-1.,1.,13.0214090879895));
#20251=CARTESIAN_POINT('',(-1.,1.,13.1555832362154));
#20252=CARTESIAN_POINT('',(-1.,-1.,13.0214090879895));
#20253=CARTESIAN_POINT('Origin',(-1.45,-1.,12.8576224825697));
#20254=CARTESIAN_POINT('',(-1.45,-1.,12.8576224825697));
#20255=CARTESIAN_POINT('',(-1.,-1.,13.0214090879895));
#20256=CARTESIAN_POINT('',(-1.45,1.,12.8576224825697));
#20257=CARTESIAN_POINT('',(-1.,1.,13.0214090879895));
#20258=CARTESIAN_POINT('',(-1.45,-1.,12.8576224825697));
#20259=CARTESIAN_POINT('Origin',(-1.45,-1.,12.6910513109172));
#20260=CARTESIAN_POINT('',(-1.45,-1.,12.6910513109172));
#20261=CARTESIAN_POINT('',(-1.45,-1.,12.8576224825697));
#20262=CARTESIAN_POINT('',(-1.45,1.,12.6910513109172));
#20263=CARTESIAN_POINT('',(-1.45,1.,12.8576224825697));
#20264=CARTESIAN_POINT('',(-1.45,-1.,12.6910513109172));
#20265=CARTESIAN_POINT('Origin',(-1.,-1.,12.5272647054974));
#20266=CARTESIAN_POINT('',(-1.,-1.,12.5272647054974));
#20267=CARTESIAN_POINT('',(-1.45,-1.,12.6910513109172));
#20268=CARTESIAN_POINT('',(-1.,1.,12.5272647054974));
#20269=CARTESIAN_POINT('',(-1.45,1.,12.6910513109172));
#20270=CARTESIAN_POINT('',(-1.,-1.,12.5272647054974));
#20271=CARTESIAN_POINT('Origin',(-1.,-1.,12.3930905572716));
#20272=CARTESIAN_POINT('',(-1.,-1.,12.3930905572716));
#20273=CARTESIAN_POINT('',(-1.,-1.,12.5272647054974));
#20274=CARTESIAN_POINT('',(-1.,1.,12.3930905572716));
#20275=CARTESIAN_POINT('',(-1.,1.,12.5272647054974));
#20276=CARTESIAN_POINT('',(-1.,-1.,12.3930905572716));
#20277=CARTESIAN_POINT('Origin',(-1.45,-1.,12.2293039518518));
#20278=CARTESIAN_POINT('',(-1.45,-1.,12.2293039518518));
#20279=CARTESIAN_POINT('',(-1.,-1.,12.3930905572716));
#20280=CARTESIAN_POINT('',(-1.45,1.,12.2293039518518));
#20281=CARTESIAN_POINT('',(-1.,1.,12.3930905572716));
#20282=CARTESIAN_POINT('',(-1.45,-1.,12.2293039518518));
#20283=CARTESIAN_POINT('Origin',(-1.45,-1.,12.0627327801993));
#20284=CARTESIAN_POINT('',(-1.45,-1.,12.0627327801993));
#20285=CARTESIAN_POINT('',(-1.45,-1.,12.2293039518518));
#20286=CARTESIAN_POINT('',(-1.45,1.,12.0627327801993));
#20287=CARTESIAN_POINT('',(-1.45,1.,12.2293039518518));
#20288=CARTESIAN_POINT('',(-1.45,-1.,12.0627327801993));
#20289=CARTESIAN_POINT('Origin',(-1.,-1.,11.8989461747795));
#20290=CARTESIAN_POINT('',(-1.,-1.,11.8989461747795));
#20291=CARTESIAN_POINT('',(-1.45,-1.,12.0627327801993));
#20292=CARTESIAN_POINT('',(-1.,1.,11.8989461747795));
#20293=CARTESIAN_POINT('',(-1.45,1.,12.0627327801993));
#20294=CARTESIAN_POINT('',(-1.,-1.,11.8989461747795));
#20295=CARTESIAN_POINT('Origin',(-1.,-1.,11.7647720265536));
#20296=CARTESIAN_POINT('',(-1.,-1.,11.7647720265536));
#20297=CARTESIAN_POINT('',(-1.,-1.,11.8989461747795));
#20298=CARTESIAN_POINT('',(-1.,1.,11.7647720265536));
#20299=CARTESIAN_POINT('',(-1.,1.,11.8989461747795));
#20300=CARTESIAN_POINT('',(-1.,-1.,11.7647720265536));
#20301=CARTESIAN_POINT('Origin',(-1.45,-1.,11.6009854211338));
#20302=CARTESIAN_POINT('',(-1.45,-1.,11.6009854211338));
#20303=CARTESIAN_POINT('',(-1.,-1.,11.7647720265536));
#20304=CARTESIAN_POINT('',(-1.45,1.,11.6009854211338));
#20305=CARTESIAN_POINT('',(-1.,1.,11.7647720265536));
#20306=CARTESIAN_POINT('',(-1.45,-1.,11.6009854211338));
#20307=CARTESIAN_POINT('Origin',(-1.45,-1.,11.4344142494813));
#20308=CARTESIAN_POINT('',(-1.45,-1.,11.4344142494813));
#20309=CARTESIAN_POINT('',(-1.45,-1.,11.6009854211338));
#20310=CARTESIAN_POINT('',(-1.45,1.,11.4344142494813));
#20311=CARTESIAN_POINT('',(-1.45,1.,11.6009854211338));
#20312=CARTESIAN_POINT('',(-1.45,-1.,11.4344142494813));
#20313=CARTESIAN_POINT('Origin',(-1.,-1.,11.2706276440615));
#20314=CARTESIAN_POINT('',(-1.,-1.,11.2706276440615));
#20315=CARTESIAN_POINT('',(-1.45,-1.,11.4344142494813));
#20316=CARTESIAN_POINT('',(-1.,1.,11.2706276440615));
#20317=CARTESIAN_POINT('',(-1.45,1.,11.4344142494813));
#20318=CARTESIAN_POINT('',(-1.,-1.,11.2706276440615));
#20319=CARTESIAN_POINT('Origin',(-1.,-1.,11.));
#20320=CARTESIAN_POINT('',(-1.,-1.,11.2706276440615));
#20321=CARTESIAN_POINT('',(-1.,1.,11.2706276440615));
#20322=CARTESIAN_POINT('Origin',(-0.625,1.,24.));
#20323=CARTESIAN_POINT('Origin',(-0.625,-1.,24.));
#20324=CARTESIAN_POINT('Origin',(1.,0.,10.8));
#20325=CARTESIAN_POINT('',(0.,-1.22464679914735E-16,40.));
#20326=CARTESIAN_POINT('Origin',(1.,0.,40.));
#20327=CARTESIAN_POINT('',(0.,-1.22464679914735E-16,10.8));
#20328=CARTESIAN_POINT('',(0.,-1.22464679914735E-16,10.8));
#20329=CARTESIAN_POINT('',(0.,-1.22464679914735E-16,10.8));
#20330=CARTESIAN_POINT('Origin',(1.,0.,10.8));
#20331=CARTESIAN_POINT('Origin',(1.,0.,40.));
#20332=CARTESIAN_POINT('Origin',(1.,0.,10.8));
#32680=UNCERTAINTY_MEASURE_WITH_UNIT(LENGTH_MEASURE(0.001),#32752,
'DISTANCE_ACCURACY_VALUE',
'Maximum model space distance between geometric entities at asserted c
onnectivities');
#32702=UNCERTAINTY_MEASURE_WITH_UNIT(LENGTH_MEASURE(0.001),#32752,
'DISTANCE_ACCURACY_VALUE',
'Maximum model space distance between geometric entities at asserted c
onnectivities');
#32729=(
GEOMETRIC_REPRESENTATION_CONTEXT(3)
GLOBAL_UNCERTAINTY_ASSIGNED_CONTEXT((#32680))
GLOBAL_UNIT_ASSIGNED_CONTEXT((#32752,#32754,#32755))
REPRESENTATION_CONTEXT('','3D')
);
#32751=(
GEOMETRIC_REPRESENTATION_CONTEXT(3)
GLOBAL_UNCERTAINTY_ASSIGNED_CONTEXT((#32702))
GLOBAL_UNIT_ASSIGNED_CONTEXT((#32752,#32754,#32755))
REPRESENTATION_CONTEXT('','3D')
);
#32752=(
LENGTH_UNIT()
NAMED_UNIT(*)
SI_UNIT(.CENTI.,.METRE.)
);
#32754=(
NAMED_UNIT(*)
PLANE_ANGLE_UNIT()
SI_UNIT($,.RADIAN.)
);
#32755=(
NAMED_UNIT(*)
SI_UNIT($,.STERADIAN.)
SOLID_ANGLE_UNIT()
);
#32782=SHAPE_DEFINITION_REPRESENTATION(#32835,#32955);
#32835=PRODUCT_DEFINITION_SHAPE('',$,#33004);
#32955=SHAPE_REPRESENTATION('',(#13567),#32729);
#32977=PRODUCT_DEFINITION_CONTEXT('part definition',#33123,'design');
#33004=PRODUCT_DEFINITION('Rack ram','Rack ram',#33052,#32977);
#33052=PRODUCT_DEFINITION_FORMATION('',$,#33151);
#33123=APPLICATION_CONTEXT(
'Core Data for Automotive Mechanical Design Process');
#33124=PRODUCT_CONTEXT('part definition',#33123,'mechanical');
#33151=PRODUCT('Rack ram','Rack ram','Rack ram',(#33124));
#33222=COLOUR_RGB('Light Blue',0.38,0.62,0.78);
#33223=FILL_AREA_STYLE_COLOUR('',#33222);
#33224=FILL_AREA_STYLE('',(#33223));
#33225=SURFACE_STYLE_FILL_AREA(#33224);
#33226=SURFACE_SIDE_STYLE('',(#33225));
#33227=SURFACE_STYLE_USAGE(.BOTH.,#33226);
#33228=PRESENTATION_STYLE_ASSIGNMENT((#33227));
ENDSEC;
END-ISO-10303-21;
